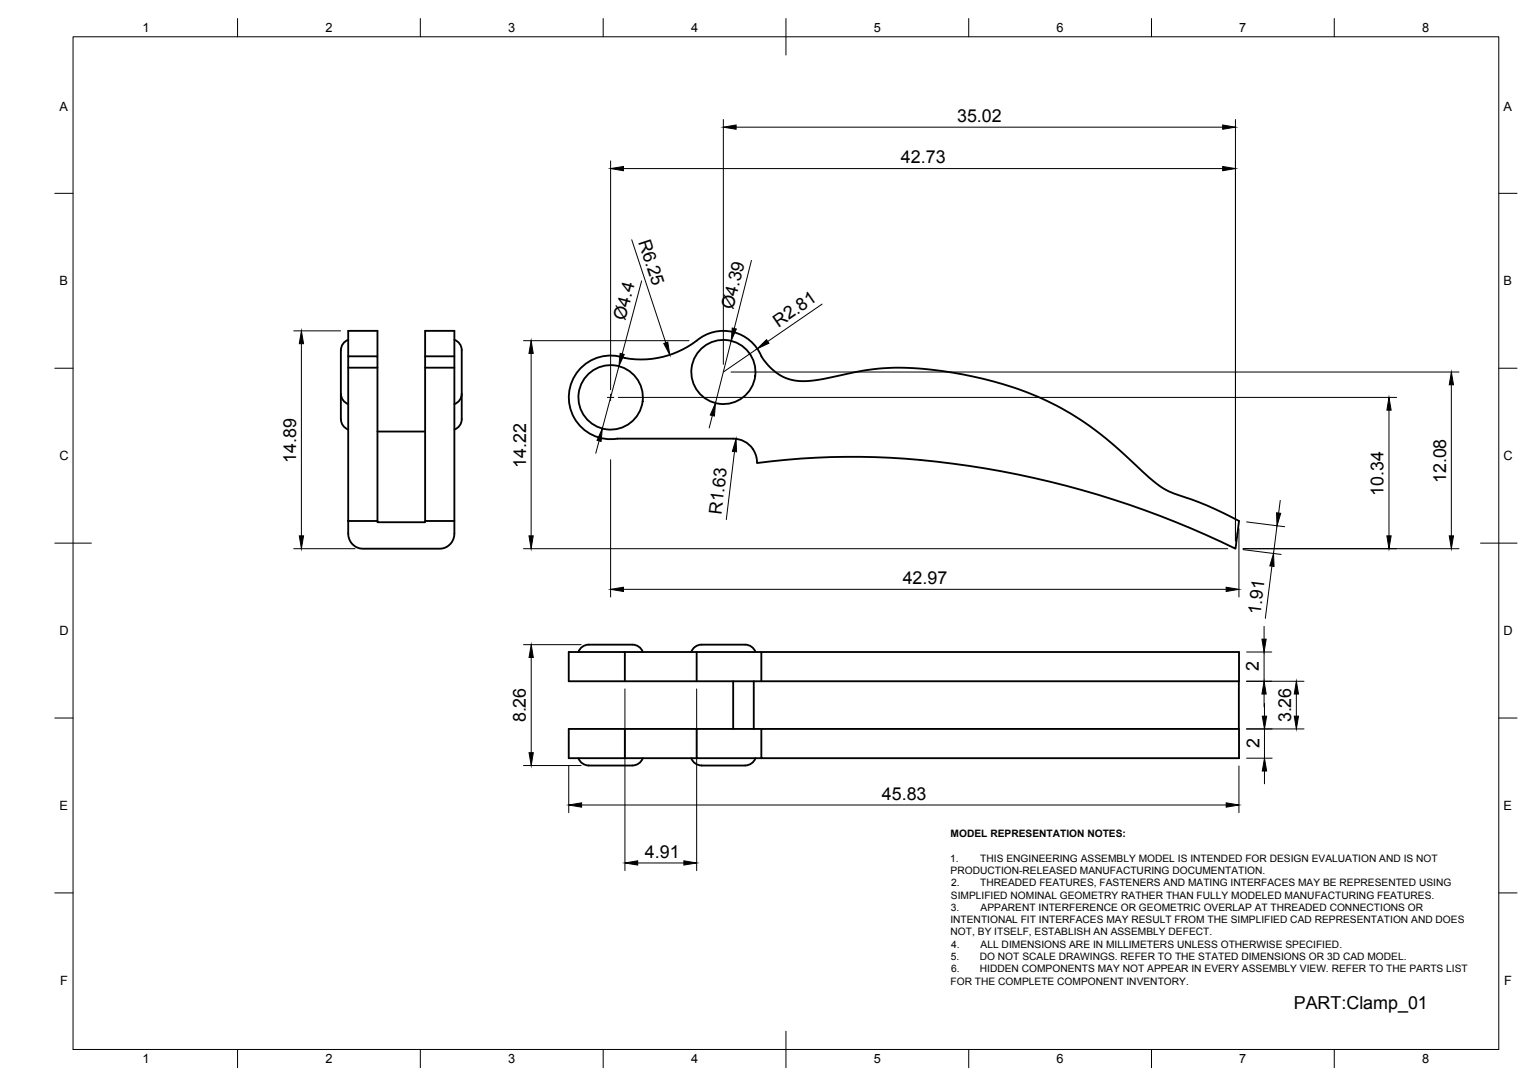
ISO-10303-21;
HEADER;
/* Generated by software containing ST-Developer
 * from STEP Tools, Inc. (www.steptools.com) 
 */

FILE_DESCRIPTION(
/* description */ (''),
/* implementation_level */ '2;1');

FILE_NAME(
/* name */ 'Clamp_01.step',
/* time_stamp */ '2026-10-05T16:20:14-07:00',
/* author */ (''),
/* organization */ (''),
/* preprocessor_version */ 'ST-DEVELOPER v20.2',
/* originating_system */ 'Autodesk Translation Framework v15.15.0.0',
/* authorisation */ '');

FILE_SCHEMA (('AUTOMOTIVE_DESIGN { 1 0 10303 214 3 1 1 }'));
ENDSEC;

DATA;
#10=MECHANICAL_DESIGN_GEOMETRIC_PRESENTATION_REPRESENTATION('',(#253),#23577);
#55=B_SPLINE_SURFACE_WITH_KNOTS('',5,1,((#21755,#21756),(#21757,#21758),
(#21759,#21760),(#21761,#21762),(#21763,#21764),(#21765,#21766),(#21767,
#21768),(#21769,#21770),(#21771,#21772),(#21773,#21774),(#21775,#21776),
(#21777,#21778),(#21779,#21780),(#21781,#21782),(#21783,#21784),(#21785,
#21786),(#21787,#21788),(#21789,#21790),(#21791,#21792),(#21793,#21794),
(#21795,#21796),(#21797,#21798),(#21799,#21800),(#21801,#21802),(#21803,
#21804),(#21805,#21806),(#21807,#21808),(#21809,#21810),(#21811,#21812),
(#21813,#21814),(#21815,#21816),(#21817,#21818),(#21819,#21820),(#21821,
#21822),(#21823,#21824),(#21825,#21826),(#21827,#21828),(#21829,#21830),
(#21831,#21832),(#21833,#21834),(#21835,#21836),(#21837,#21838),(#21839,
#21840),(#21841,#21842),(#21843,#21844),(#21845,#21846),(#21847,#21848),
(#21849,#21850),(#21851,#21852),(#21853,#21854),(#21855,#21856),(#21857,
#21858),(#21859,#21860),(#21861,#21862),(#21863,#21864)),.UNSPECIFIED.,
 .F.,.F.,.F.,(6,1,1,1,1,1,1,1,1,1,1,1,1,1,1,1,1,1,1,1,1,1,1,1,1,1,1,1,1,
1,1,1,1,1,1,1,1,1,1,1,1,1,1,1,1,1,1,1,1,1,6),(2,2),(0.,0.02,0.04,0.06,0.08,
0.1,0.12,0.14,0.16,0.18,0.2,0.22,0.24,0.26,0.28,0.3,0.32,0.34,0.36,0.38,
0.4,0.42,0.44,0.46,0.48,0.5,0.52,0.54,0.56,0.58,0.6,0.62,0.64,0.66,0.68,
0.7,0.72,0.74,0.76,0.78,0.8,0.82,0.84,0.86,0.88,0.9,0.92,0.940000000000001,
0.960000000000001,0.980000000000001,0.99866513431215),(0.,0.24),
 .UNSPECIFIED.);
#56=B_SPLINE_SURFACE_WITH_KNOTS('',5,1,((#22096,#22097),(#22098,#22099),
(#22100,#22101),(#22102,#22103),(#22104,#22105),(#22106,#22107),(#22108,
#22109),(#22110,#22111),(#22112,#22113),(#22114,#22115),(#22116,#22117),
(#22118,#22119),(#22120,#22121),(#22122,#22123),(#22124,#22125),(#22126,
#22127),(#22128,#22129),(#22130,#22131),(#22132,#22133),(#22134,#22135),
(#22136,#22137),(#22138,#22139),(#22140,#22141),(#22142,#22143),(#22144,
#22145),(#22146,#22147),(#22148,#22149),(#22150,#22151),(#22152,#22153),
(#22154,#22155),(#22156,#22157),(#22158,#22159),(#22160,#22161),(#22162,
#22163),(#22164,#22165),(#22166,#22167),(#22168,#22169),(#22170,#22171),
(#22172,#22173),(#22174,#22175),(#22176,#22177),(#22178,#22179),(#22180,
#22181),(#22182,#22183),(#22184,#22185),(#22186,#22187),(#22188,#22189),
(#22190,#22191),(#22192,#22193),(#22194,#22195),(#22196,#22197),(#22198,
#22199),(#22200,#22201),(#22202,#22203),(#22204,#22205)),.UNSPECIFIED.,
 .F.,.F.,.F.,(6,1,1,1,1,1,1,1,1,1,1,1,1,1,1,1,1,1,1,1,1,1,1,1,1,1,1,1,1,
1,1,1,1,1,1,1,1,1,1,1,1,1,1,1,1,1,1,1,1,1,6),(2,2),(0.,0.02,0.04,0.06,0.08,
0.1,0.12,0.14,0.16,0.18,0.2,0.22,0.24,0.26,0.28,0.3,0.32,0.34,0.36,0.38,
0.4,0.42,0.44,0.46,0.48,0.5,0.52,0.54,0.56,0.58,0.6,0.62,0.64,0.66,0.68,
0.7,0.72,0.74,0.76,0.78,0.8,0.82,0.84,0.86,0.88,0.9,0.92,0.940000000000001,
0.960000000000001,0.980000000000001,0.99866513431215),(0.,0.24),
 .UNSPECIFIED.);
#173=B_SPLINE_CURVE_WITH_KNOTS('',3,(#21553,#21554,#21555,#21556,#21557,
#21558,#21559,#21560,#21561,#21562),.UNSPECIFIED.,.F.,.F.,(4,2,2,2,4),(0.304370745831088,
0.340749860871315,0.378176848018549,0.416877357705943,0.456616383722292),
 .UNSPECIFIED.);
#174=B_SPLINE_CURVE_WITH_KNOTS('',3,(#21571,#21572,#21573,#21574,#21575,
#21576,#21577,#21578,#21579,#21580,#21581,#21582),.UNSPECIFIED.,.F.,.F.,
(4,2,2,2,2,4),(-0.956034309409163,-0.919797905610199,-0.883592147057887,
-0.844404551538294,-0.805088366243444,-0.793069564297015),.UNSPECIFIED.);
#175=B_SPLINE_CURVE_WITH_KNOTS('',3,(#21606,#21607,#21608,#21609,#21610,
#21611,#21612,#21613,#21614,#21615,#21616,#21617),.UNSPECIFIED.,.F.,.F.,
(4,2,2,2,2,4),(-0.793069564419585,-0.765429318917777,-0.726356329910807,
-0.690453978752587,-0.655278338273468,-0.628541412295733),.UNSPECIFIED.);
#176=B_SPLINE_CURVE_WITH_KNOTS('',3,(#21620,#21621,#21622,#21623,#21624,
#21625,#21626,#21627,#21628,#21629),.UNSPECIFIED.,.F.,.F.,(4,2,2,2,4),(0.152125107939884,
0.191864133956234,0.230564643643628,0.267991630790861,0.304370745831088),
 .UNSPECIFIED.);
#177=B_SPLINE_CURVE_WITH_KNOTS('',5,(#21645,#21646,#21647,#21648,#21649,
#21650,#21651,#21652,#21653,#21654,#21655,#21656,#21657,#21658,#21659,#21660,
#21661,#21662,#21663,#21664,#21665,#21666,#21667,#21668,#21669,#21670,#21671,
#21672,#21673,#21674,#21675,#21676,#21677,#21678,#21679,#21680,#21681,#21682,
#21683,#21684,#21685,#21686,#21687,#21688,#21689,#21690,#21691,#21692,#21693,
#21694,#21695,#21696,#21697,#21698,#21699),.UNSPECIFIED.,.F.,.F.,(6,1,1,
1,1,1,1,1,1,1,1,1,1,1,1,1,1,1,1,1,1,1,1,1,1,1,1,1,1,1,1,1,1,1,1,1,1,1,1,
1,1,1,1,1,1,1,1,1,1,1,6),(0.,0.02,0.04,0.06,0.08,0.1,0.12,0.14,0.16,0.18,
0.2,0.22,0.24,0.26,0.28,0.3,0.32,0.34,0.36,0.38,0.4,0.42,0.44,0.46,0.48,
0.5,0.52,0.54,0.56,0.58,0.6,0.62,0.64,0.66,0.68,0.7,0.72,0.74,0.76,0.78,
0.8,0.82,0.84,0.86,0.88,0.9,0.92,0.940000000000001,0.960000000000001,0.980000000000001,
0.99866513431215),.UNSPECIFIED.);
#178=B_SPLINE_CURVE_WITH_KNOTS('',5,(#21867,#21868,#21869,#21870,#21871,
#21872,#21873,#21874,#21875,#21876,#21877,#21878,#21879,#21880,#21881,#21882,
#21883,#21884,#21885,#21886,#21887,#21888,#21889,#21890,#21891,#21892,#21893,
#21894,#21895,#21896,#21897,#21898,#21899,#21900,#21901,#21902,#21903,#21904,
#21905,#21906,#21907,#21908,#21909,#21910,#21911,#21912,#21913,#21914,#21915,
#21916,#21917,#21918,#21919,#21920,#21921),.UNSPECIFIED.,.F.,.F.,(6,1,1,
1,1,1,1,1,1,1,1,1,1,1,1,1,1,1,1,1,1,1,1,1,1,1,1,1,1,1,1,1,1,1,1,1,1,1,1,
1,1,1,1,1,1,1,1,1,1,1,6),(0.,0.02,0.04,0.06,0.08,0.1,0.12,0.14,0.16,0.18,
0.2,0.22,0.24,0.26,0.28,0.3,0.32,0.34,0.36,0.38,0.4,0.42,0.44,0.46,0.48,
0.5,0.52,0.54,0.56,0.58,0.6,0.62,0.64,0.66,0.68,0.7,0.72,0.74,0.76,0.78,
0.8,0.82,0.84,0.86,0.88,0.9,0.92,0.940000000000001,0.960000000000001,0.980000000000001,
0.998665134312151),.UNSPECIFIED.);
#179=B_SPLINE_CURVE_WITH_KNOTS('',5,(#21925,#21926,#21927,#21928,#21929,
#21930,#21931,#21932,#21933,#21934,#21935,#21936,#21937,#21938,#21939,#21940,
#21941,#21942,#21943,#21944,#21945,#21946,#21947,#21948,#21949,#21950,#21951,
#21952,#21953,#21954,#21955,#21956,#21957,#21958,#21959,#21960,#21961,#21962,
#21963,#21964,#21965,#21966,#21967,#21968,#21969,#21970,#21971,#21972,#21973,
#21974,#21975,#21976,#21977,#21978,#21979),.UNSPECIFIED.,.F.,.F.,(6,1,1,
1,1,1,1,1,1,1,1,1,1,1,1,1,1,1,1,1,1,1,1,1,1,1,1,1,1,1,1,1,1,1,1,1,1,1,1,
1,1,1,1,1,1,1,1,1,1,1,6),(0.,0.02,0.04,0.06,0.08,0.1,0.12,0.14,0.16,0.18,
0.2,0.22,0.24,0.26,0.28,0.3,0.32,0.34,0.36,0.38,0.4,0.42,0.44,0.46,0.48,
0.5,0.52,0.54,0.56,0.58,0.6,0.62,0.64,0.66,0.68,0.7,0.72,0.74,0.76,0.78,
0.8,0.82,0.84,0.86,0.88,0.9,0.92,0.940000000000001,0.960000000000001,0.980000000000001,
0.99866513431215),.UNSPECIFIED.);
#180=B_SPLINE_CURVE_WITH_KNOTS('',5,(#22022,#22023,#22024,#22025,#22026,
#22027,#22028,#22029,#22030,#22031,#22032,#22033,#22034,#22035,#22036,#22037,
#22038,#22039,#22040,#22041,#22042,#22043,#22044,#22045,#22046,#22047,#22048,
#22049,#22050,#22051,#22052,#22053,#22054,#22055,#22056,#22057,#22058,#22059,
#22060,#22061,#22062,#22063,#22064,#22065,#22066,#22067,#22068,#22069,#22070,
#22071,#22072,#22073,#22074,#22075,#22076),.UNSPECIFIED.,.F.,.F.,(6,1,1,
1,1,1,1,1,1,1,1,1,1,1,1,1,1,1,1,1,1,1,1,1,1,1,1,1,1,1,1,1,1,1,1,1,1,1,1,
1,1,1,1,1,1,1,1,1,1,1,6),(0.,0.02,0.04,0.06,0.08,0.1,0.12,0.14,0.16,0.18,
0.2,0.22,0.24,0.26,0.28,0.3,0.32,0.34,0.36,0.38,0.4,0.42,0.44,0.46,0.48,
0.5,0.52,0.54,0.56,0.58,0.6,0.62,0.64,0.66,0.68,0.7,0.72,0.74,0.76,0.78,
0.8,0.82,0.84,0.86,0.88,0.9,0.92,0.940000000000001,0.960000000000001,0.980000000000001,
0.998665134312151),.UNSPECIFIED.);
#217=TOROIDAL_SURFACE('',#4486,63.3332952479771,1.);
#218=TOROIDAL_SURFACE('',#4490,50.7730300598816,1.);
#219=TOROIDAL_SURFACE('',#4500,63.3332952479771,1.);
#220=TOROIDAL_SURFACE('',#4503,50.7730300598816,1.);
#221=TOROIDAL_SURFACE('',#4513,1.49422838778107,0.75);
#222=TOROIDAL_SURFACE('',#4519,1.48767572173512,0.75);
#223=TOROIDAL_SURFACE('',#4525,1.49422838778107,0.75);
#224=TOROIDAL_SURFACE('',#4532,1.48767572173512,0.75);
#235=SHAPE_REPRESENTATION_RELATIONSHIP('SRR','None',#23618,#244);
#244=ADVANCED_BREP_SHAPE_REPRESENTATION('',(#262),#23574);
#253=STYLED_ITEM('',(#23668),#262);
#262=MANIFOLD_SOLID_BREP('Body1',#4163);
#286=FACE_BOUND('',#778,.T.);
#287=FACE_BOUND('',#779,.T.);
#288=FACE_BOUND('',#800,.T.);
#289=FACE_BOUND('',#801,.T.);
#290=FACE_BOUND('',#803,.T.);
#291=FACE_BOUND('',#804,.T.);
#292=FACE_BOUND('',#809,.T.);
#293=FACE_BOUND('',#810,.T.);
#361=PLANE('',#4505);
#362=PLANE('',#4511);
#363=PLANE('',#4516);
#364=PLANE('',#4517);
#365=PLANE('',#4522);
#366=PLANE('',#4523);
#367=PLANE('',#4529);
#368=PLANE('',#4530);
#369=PLANE('',#4536);
#370=PLANE('',#4541);
#371=PLANE('',#4551);
#372=PLANE('',#4552);
#373=PLANE('',#4555);
#374=PLANE('',#4560);
#375=PLANE('',#4568);
#376=PLANE('',#4569);
#523=FACE_OUTER_BOUND('',#770,.T.);
#524=FACE_OUTER_BOUND('',#771,.T.);
#525=FACE_OUTER_BOUND('',#772,.T.);
#526=FACE_OUTER_BOUND('',#773,.T.);
#527=FACE_OUTER_BOUND('',#774,.T.);
#528=FACE_OUTER_BOUND('',#775,.T.);
#529=FACE_OUTER_BOUND('',#776,.T.);
#530=FACE_OUTER_BOUND('',#777,.T.);
#531=FACE_OUTER_BOUND('',#780,.T.);
#532=FACE_OUTER_BOUND('',#781,.T.);
#533=FACE_OUTER_BOUND('',#782,.T.);
#534=FACE_OUTER_BOUND('',#783,.T.);
#535=FACE_OUTER_BOUND('',#784,.T.);
#536=FACE_OUTER_BOUND('',#785,.T.);
#537=FACE_OUTER_BOUND('',#786,.T.);
#538=FACE_OUTER_BOUND('',#787,.T.);
#539=FACE_OUTER_BOUND('',#788,.T.);
#540=FACE_OUTER_BOUND('',#789,.T.);
#541=FACE_OUTER_BOUND('',#790,.T.);
#542=FACE_OUTER_BOUND('',#791,.T.);
#543=FACE_OUTER_BOUND('',#792,.T.);
#544=FACE_OUTER_BOUND('',#793,.T.);
#545=FACE_OUTER_BOUND('',#794,.T.);
#546=FACE_OUTER_BOUND('',#795,.T.);
#547=FACE_OUTER_BOUND('',#796,.T.);
#548=FACE_OUTER_BOUND('',#797,.T.);
#549=FACE_OUTER_BOUND('',#798,.T.);
#550=FACE_OUTER_BOUND('',#799,.T.);
#551=FACE_OUTER_BOUND('',#802,.T.);
#552=FACE_OUTER_BOUND('',#805,.T.);
#553=FACE_OUTER_BOUND('',#806,.T.);
#554=FACE_OUTER_BOUND('',#807,.T.);
#555=FACE_OUTER_BOUND('',#808,.T.);
#556=FACE_OUTER_BOUND('',#811,.T.);
#557=FACE_OUTER_BOUND('',#812,.T.);
#558=FACE_OUTER_BOUND('',#813,.T.);
#559=FACE_OUTER_BOUND('',#814,.T.);
#560=FACE_OUTER_BOUND('',#815,.T.);
#561=FACE_OUTER_BOUND('',#816,.T.);
#562=FACE_OUTER_BOUND('',#817,.T.);
#563=FACE_OUTER_BOUND('',#818,.T.);
#770=EDGE_LOOP('',(#3387,#3388,#3389,#3390));
#771=EDGE_LOOP('',(#3391,#3392,#3393,#3394));
#772=EDGE_LOOP('',(#3395,#3396,#3397,#3398));
#773=EDGE_LOOP('',(#3399,#3400,#3401,#3402));
#774=EDGE_LOOP('',(#3403,#3404,#3405,#3406,#3407,#3408,#3409,#3410));
#775=EDGE_LOOP('',(#3411,#3412,#3413,#3414));
#776=EDGE_LOOP('',(#3415,#3416,#3417,#3418));
#777=EDGE_LOOP('',(#3419,#3420,#3421,#3422,#3423,#3424,#3425,#3426,#3427));
#778=EDGE_LOOP('',(#3428));
#779=EDGE_LOOP('',(#3429));
#780=EDGE_LOOP('',(#3430));
#781=EDGE_LOOP('',(#3431,#3432,#3433,#3434));
#782=EDGE_LOOP('',(#3435));
#783=EDGE_LOOP('',(#3436));
#784=EDGE_LOOP('',(#3437,#3438,#3439,#3440));
#785=EDGE_LOOP('',(#3441));
#786=EDGE_LOOP('',(#3442));
#787=EDGE_LOOP('',(#3443,#3444,#3445,#3446));
#788=EDGE_LOOP('',(#3447));
#789=EDGE_LOOP('',(#3448));
#790=EDGE_LOOP('',(#3449,#3450,#3451,#3452));
#791=EDGE_LOOP('',(#3453));
#792=EDGE_LOOP('',(#3454,#3455,#3456,#3457));
#793=EDGE_LOOP('',(#3458,#3459,#3460,#3461));
#794=EDGE_LOOP('',(#3462,#3463,#3464,#3465));
#795=EDGE_LOOP('',(#3466,#3467,#3468,#3469));
#796=EDGE_LOOP('',(#3470,#3471,#3472,#3473));
#797=EDGE_LOOP('',(#3474,#3475,#3476,#3477));
#798=EDGE_LOOP('',(#3478,#3479,#3480,#3481));
#799=EDGE_LOOP('',(#3482,#3483,#3484,#3485,#3486,#3487,#3488,#3489,#3490));
#800=EDGE_LOOP('',(#3491));
#801=EDGE_LOOP('',(#3492));
#802=EDGE_LOOP('',(#3493,#3494,#3495,#3496,#3497,#3498,#3499,#3500,#3501));
#803=EDGE_LOOP('',(#3502));
#804=EDGE_LOOP('',(#3503));
#805=EDGE_LOOP('',(#3504,#3505,#3506,#3507));
#806=EDGE_LOOP('',(#3508,#3509,#3510,#3511));
#807=EDGE_LOOP('',(#3512,#3513,#3514,#3515));
#808=EDGE_LOOP('',(#3516,#3517,#3518,#3519,#3520,#3521,#3522,#3523,#3524));
#809=EDGE_LOOP('',(#3525));
#810=EDGE_LOOP('',(#3526));
#811=EDGE_LOOP('',(#3527,#3528,#3529,#3530));
#812=EDGE_LOOP('',(#3531,#3532,#3533,#3534));
#813=EDGE_LOOP('',(#3535,#3536,#3537,#3538));
#814=EDGE_LOOP('',(#3539,#3540,#3541,#3542,#3543,#3544,#3545,#3546,#3547,
#3548));
#815=EDGE_LOOP('',(#3549,#3550,#3551,#3552));
#816=EDGE_LOOP('',(#3553,#3554,#3555,#3556));
#817=EDGE_LOOP('',(#3557,#3558,#3559,#3560));
#818=EDGE_LOOP('',(#3561,#3562,#3563,#3564));
#1069=LINE('',#21587,#1354);
#1070=LINE('',#21590,#1355);
#1071=LINE('',#21593,#1356);
#1072=LINE('',#21599,#1357);
#1073=LINE('',#21601,#1358);
#1074=LINE('',#21603,#1359);
#1075=LINE('',#21637,#1360);
#1076=LINE('',#21700,#1361);
#1077=LINE('',#21743,#1362);
#1078=LINE('',#21747,#1363);
#1079=LINE('',#21751,#1364);
#1080=LINE('',#21753,#1365);
#1081=LINE('',#21754,#1366);
#1082=LINE('',#21923,#1367);
#1083=LINE('',#21980,#1368);
#1084=LINE('',#21985,#1369);
#1085=LINE('',#21991,#1370);
#1086=LINE('',#21997,#1371);
#1087=LINE('',#22000,#1372);
#1088=LINE('',#22002,#1373);
#1089=LINE('',#22008,#1374);
#1090=LINE('',#22009,#1375);
#1091=LINE('',#22012,#1376);
#1092=LINE('',#22016,#1377);
#1093=LINE('',#22020,#1378);
#1094=LINE('',#22083,#1379);
#1095=LINE('',#22089,#1380);
#1096=LINE('',#22091,#1381);
#1097=LINE('',#22093,#1382);
#1098=LINE('',#22095,#1383);
#1099=LINE('',#22206,#1384);
#1100=LINE('',#22208,#1385);
#1101=LINE('',#22210,#1386);
#1354=VECTOR('',#5316,10.);
#1355=VECTOR('',#5319,10.);
#1356=VECTOR('',#5322,10.);
#1357=VECTOR('',#5329,10.);
#1358=VECTOR('',#5330,10.);
#1359=VECTOR('',#5331,10.);
#1360=VECTOR('',#5346,10.);
#1361=VECTOR('',#5353,10.);
#1362=VECTOR('',#5412,1.69478250292167);
#1363=VECTOR('',#5417,1.70133516896762);
#1364=VECTOR('',#5422,10.);
#1365=VECTOR('',#5423,10.);
#1366=VECTOR('',#5424,10.);
#1367=VECTOR('',#5425,10.);
#1368=VECTOR('',#5426,10.);
#1369=VECTOR('',#5431,10.);
#1370=VECTOR('',#5438,10.);
#1371=VECTOR('',#5449,10.);
#1372=VECTOR('',#5452,10.);
#1373=VECTOR('',#5453,10.);
#1374=VECTOR('',#5460,10.);
#1375=VECTOR('',#5461,10.);
#1376=VECTOR('',#5464,10.);
#1377=VECTOR('',#5469,10.);
#1378=VECTOR('',#5474,10.);
#1379=VECTOR('',#5481,10.);
#1380=VECTOR('',#5488,1.69478250292167);
#1381=VECTOR('',#5491,1.70133516896762);
#1382=VECTOR('',#5494,10.);
#1383=VECTOR('',#5497,10.);
#1384=VECTOR('',#5498,10.);
#1385=VECTOR('',#5501,10.);
#1386=VECTOR('',#5504,10.);
#1536=CIRCLE('',#4487,63.3332952479771);
#1537=CIRCLE('',#4488,1.);
#1538=CIRCLE('',#4489,62.3332952479771);
#1539=CIRCLE('',#4491,49.7730300598817);
#1540=CIRCLE('',#4492,50.7730300598817);
#1541=CIRCLE('',#4494,62.3332952479771);
#1542=CIRCLE('',#4496,49.7730300598817);
#1543=CIRCLE('',#4498,1.6332945980533);
#1544=CIRCLE('',#4499,1.6332945980533);
#1545=CIRCLE('',#4501,1.);
#1546=CIRCLE('',#4502,63.3332952479771);
#1547=CIRCLE('',#4504,50.7730300598817);
#1548=CIRCLE('',#4506,2.8615696413584);
#1549=CIRCLE('',#4507,6.2515148621032);
#1550=CIRCLE('',#4508,2.81236096609945);
#1551=CIRCLE('',#4509,2.19478250292167);
#1552=CIRCLE('',#4510,2.20133516896762);
#1553=CIRCLE('',#4512,1.70133516896762);
#1554=CIRCLE('',#4514,1.49422838778107);
#1555=CIRCLE('',#4515,0.75);
#1556=CIRCLE('',#4518,1.69478250292167);
#1557=CIRCLE('',#4520,1.48767572173512);
#1558=CIRCLE('',#4521,0.75);
#1559=CIRCLE('',#4524,1.70133516896762);
#1560=CIRCLE('',#4526,1.49422838778107);
#1561=CIRCLE('',#4527,0.75);
#1562=CIRCLE('',#4528,2.20133516896762);
#1563=CIRCLE('',#4531,1.69478250292167);
#1564=CIRCLE('',#4533,1.48767572173512);
#1565=CIRCLE('',#4534,0.75);
#1566=CIRCLE('',#4535,2.19478250292167);
#1567=CIRCLE('',#4538,1.69478250292167);
#1568=CIRCLE('',#4540,1.70133516896762);
#1569=CIRCLE('',#4543,2.81236096609945);
#1570=CIRCLE('',#4544,2.81236096609945);
#1571=CIRCLE('',#4546,6.2515148621032);
#1572=CIRCLE('',#4547,6.2515148621032);
#1573=CIRCLE('',#4549,2.8615696413584);
#1574=CIRCLE('',#4550,2.8615696413584);
#1575=CIRCLE('',#4553,64.0604216491307);
#1576=CIRCLE('',#4554,51.5001564610352);
#1577=CIRCLE('',#4557,51.5001564610352);
#1578=CIRCLE('',#4559,64.0604216491307);
#1579=CIRCLE('',#4561,2.81236096609945);
#1580=CIRCLE('',#4562,6.2515148621032);
#1581=CIRCLE('',#4563,2.8615696413584);
#1582=CIRCLE('',#4564,1.69478250292167);
#1583=CIRCLE('',#4565,1.70133516896762);
#1893=VERTEX_POINT('',#21551);
#1894=VERTEX_POINT('',#21552);
#1895=VERTEX_POINT('',#21563);
#1896=VERTEX_POINT('',#21565);
#1897=VERTEX_POINT('',#21569);
#1898=VERTEX_POINT('',#21570);
#1899=VERTEX_POINT('',#21586);
#1900=VERTEX_POINT('',#21588);
#1901=VERTEX_POINT('',#21592);
#1902=VERTEX_POINT('',#21596);
#1903=VERTEX_POINT('',#21598);
#1904=VERTEX_POINT('',#21600);
#1905=VERTEX_POINT('',#21602);
#1906=VERTEX_POINT('',#21604);
#1907=VERTEX_POINT('',#21619);
#1908=VERTEX_POINT('',#21630);
#1909=VERTEX_POINT('',#21636);
#1910=VERTEX_POINT('',#21638);
#1911=VERTEX_POINT('',#21640);
#1912=VERTEX_POINT('',#21642);
#1913=VERTEX_POINT('',#21644);
#1914=VERTEX_POINT('',#21701);
#1915=VERTEX_POINT('',#21703);
#1916=VERTEX_POINT('',#21706);
#1917=VERTEX_POINT('',#21709);
#1918=VERTEX_POINT('',#21714);
#1919=VERTEX_POINT('',#21717);
#1920=VERTEX_POINT('',#21722);
#1921=VERTEX_POINT('',#21725);
#1922=VERTEX_POINT('',#21727);
#1923=VERTEX_POINT('',#21732);
#1924=VERTEX_POINT('',#21735);
#1925=VERTEX_POINT('',#21737);
#1926=VERTEX_POINT('',#21742);
#1927=VERTEX_POINT('',#21746);
#1928=VERTEX_POINT('',#21750);
#1929=VERTEX_POINT('',#21752);
#1930=VERTEX_POINT('',#21865);
#1931=VERTEX_POINT('',#21866);
#1932=VERTEX_POINT('',#21922);
#1933=VERTEX_POINT('',#21924);
#1934=VERTEX_POINT('',#21982);
#1935=VERTEX_POINT('',#21984);
#1936=VERTEX_POINT('',#21988);
#1937=VERTEX_POINT('',#21990);
#1938=VERTEX_POINT('',#21999);
#1939=VERTEX_POINT('',#22001);
#1940=VERTEX_POINT('',#22003);
#1941=VERTEX_POINT('',#22007);
#1942=VERTEX_POINT('',#22011);
#1943=VERTEX_POINT('',#22015);
#1944=VERTEX_POINT('',#22019);
#1945=VERTEX_POINT('',#22021);
#1946=VERTEX_POINT('',#22077);
#1947=VERTEX_POINT('',#22079);
#1948=VERTEX_POINT('',#22081);
#1949=VERTEX_POINT('',#22084);
#1950=VERTEX_POINT('',#22086);
#2410=EDGE_CURVE('',#1893,#1894,#173,.T.);
#2411=EDGE_CURVE('',#1894,#1895,#1536,.T.);
#2412=EDGE_CURVE('',#1895,#1896,#1537,.T.);
#2413=EDGE_CURVE('',#1896,#1893,#1538,.T.);
#2414=EDGE_CURVE('',#1897,#1898,#174,.T.);
#2415=EDGE_CURVE('',#1898,#1896,#1539,.T.);
#2416=EDGE_CURVE('',#1895,#1897,#1540,.T.);
#2417=EDGE_CURVE('',#1896,#1899,#1069,.T.);
#2418=EDGE_CURVE('',#1900,#1899,#1541,.T.);
#2419=EDGE_CURVE('',#1893,#1900,#1070,.T.);
#2420=EDGE_CURVE('',#1898,#1901,#1071,.T.);
#2421=EDGE_CURVE('',#1899,#1901,#1542,.T.);
#2422=EDGE_CURVE('',#1897,#1902,#1543,.T.);
#2423=EDGE_CURVE('',#1903,#1902,#1072,.T.);
#2424=EDGE_CURVE('',#1904,#1903,#1073,.T.);
#2425=EDGE_CURVE('',#1904,#1905,#1074,.T.);
#2426=EDGE_CURVE('',#1906,#1905,#1544,.T.);
#2427=EDGE_CURVE('',#1901,#1906,#175,.T.);
#2428=EDGE_CURVE('',#1907,#1900,#176,.T.);
#2429=EDGE_CURVE('',#1899,#1908,#1545,.T.);
#2430=EDGE_CURVE('',#1908,#1907,#1546,.T.);
#2431=EDGE_CURVE('',#1906,#1908,#1547,.T.);
#2432=EDGE_CURVE('',#1905,#1909,#1075,.T.);
#2433=EDGE_CURVE('',#1909,#1910,#1548,.T.);
#2434=EDGE_CURVE('',#1910,#1911,#1549,.T.);
#2435=EDGE_CURVE('',#1911,#1912,#1550,.T.);
#2436=EDGE_CURVE('',#1912,#1913,#177,.T.);
#2437=EDGE_CURVE('',#1913,#1907,#1076,.T.);
#2438=EDGE_CURVE('',#1914,#1914,#1551,.T.);
#2439=EDGE_CURVE('',#1915,#1915,#1552,.T.);
#2440=EDGE_CURVE('',#1916,#1916,#1553,.T.);
#2441=EDGE_CURVE('',#1917,#1917,#1554,.T.);
#2442=EDGE_CURVE('',#1917,#1915,#1555,.T.);
#2443=EDGE_CURVE('',#1918,#1918,#1556,.T.);
#2444=EDGE_CURVE('',#1919,#1919,#1557,.T.);
#2445=EDGE_CURVE('',#1919,#1914,#1558,.T.);
#2446=EDGE_CURVE('',#1920,#1920,#1559,.T.);
#2447=EDGE_CURVE('',#1921,#1921,#1560,.T.);
#2448=EDGE_CURVE('',#1921,#1922,#1561,.T.);
#2449=EDGE_CURVE('',#1922,#1922,#1562,.T.);
#2450=EDGE_CURVE('',#1923,#1923,#1563,.T.);
#2451=EDGE_CURVE('',#1924,#1924,#1564,.T.);
#2452=EDGE_CURVE('',#1924,#1925,#1565,.T.);
#2453=EDGE_CURVE('',#1925,#1925,#1566,.T.);
#2454=EDGE_CURVE('',#1923,#1926,#1077,.T.);
#2455=EDGE_CURVE('',#1926,#1926,#1567,.T.);
#2456=EDGE_CURVE('',#1920,#1927,#1078,.T.);
#2457=EDGE_CURVE('',#1927,#1927,#1568,.T.);
#2458=EDGE_CURVE('',#1928,#1903,#1079,.T.);
#2459=EDGE_CURVE('',#1902,#1929,#1080,.T.);
#2460=EDGE_CURVE('',#1928,#1929,#1081,.T.);
#2461=EDGE_CURVE('',#1930,#1931,#178,.T.);
#2462=EDGE_CURVE('',#1930,#1932,#1082,.T.);
#2463=EDGE_CURVE('',#1932,#1933,#179,.T.);
#2464=EDGE_CURVE('',#1931,#1933,#1083,.T.);
#2465=EDGE_CURVE('',#1934,#1930,#1569,.T.);
#2466=EDGE_CURVE('',#1934,#1935,#1084,.T.);
#2467=EDGE_CURVE('',#1935,#1932,#1570,.T.);
#2468=EDGE_CURVE('',#1934,#1936,#1571,.T.);
#2469=EDGE_CURVE('',#1936,#1937,#1085,.T.);
#2470=EDGE_CURVE('',#1937,#1935,#1572,.T.);
#2471=EDGE_CURVE('',#1928,#1936,#1573,.T.);
#2472=EDGE_CURVE('',#1929,#1937,#1574,.T.);
#2473=EDGE_CURVE('',#1933,#1894,#1086,.T.);
#2474=EDGE_CURVE('',#1903,#1938,#1087,.T.);
#2475=EDGE_CURVE('',#1939,#1931,#1088,.T.);
#2476=EDGE_CURVE('',#1940,#1939,#1575,.T.);
#2477=EDGE_CURVE('',#1938,#1940,#1576,.T.);
#2478=EDGE_CURVE('',#1941,#1938,#1089,.T.);
#2479=EDGE_CURVE('',#1904,#1941,#1090,.T.);
#2480=EDGE_CURVE('',#1942,#1940,#1091,.T.);
#2481=EDGE_CURVE('',#1941,#1942,#1577,.T.);
#2482=EDGE_CURVE('',#1943,#1939,#1092,.T.);
#2483=EDGE_CURVE('',#1942,#1943,#1578,.T.);
#2484=EDGE_CURVE('',#1943,#1944,#1093,.T.);
#2485=EDGE_CURVE('',#1945,#1944,#180,.T.);
#2486=EDGE_CURVE('',#1946,#1945,#1579,.T.);
#2487=EDGE_CURVE('',#1946,#1947,#1580,.T.);
#2488=EDGE_CURVE('',#1948,#1947,#1581,.T.);
#2489=EDGE_CURVE('',#1948,#1904,#1094,.T.);
#2490=EDGE_CURVE('',#1949,#1949,#1582,.T.);
#2491=EDGE_CURVE('',#1950,#1950,#1583,.T.);
#2492=EDGE_CURVE('',#1949,#1918,#1095,.T.);
#2493=EDGE_CURVE('',#1950,#1916,#1096,.T.);
#2494=EDGE_CURVE('',#1948,#1909,#1097,.T.);
#2495=EDGE_CURVE('',#1944,#1913,#1098,.T.);
#2496=EDGE_CURVE('',#1945,#1912,#1099,.T.);
#2497=EDGE_CURVE('',#1946,#1911,#1100,.T.);
#2498=EDGE_CURVE('',#1947,#1910,#1101,.T.);
#3387=ORIENTED_EDGE('',*,*,#2410,.T.);
#3388=ORIENTED_EDGE('',*,*,#2411,.T.);
#3389=ORIENTED_EDGE('',*,*,#2412,.T.);
#3390=ORIENTED_EDGE('',*,*,#2413,.T.);
#3391=ORIENTED_EDGE('',*,*,#2414,.T.);
#3392=ORIENTED_EDGE('',*,*,#2415,.T.);
#3393=ORIENTED_EDGE('',*,*,#2412,.F.);
#3394=ORIENTED_EDGE('',*,*,#2416,.T.);
#3395=ORIENTED_EDGE('',*,*,#2413,.F.);
#3396=ORIENTED_EDGE('',*,*,#2417,.T.);
#3397=ORIENTED_EDGE('',*,*,#2418,.F.);
#3398=ORIENTED_EDGE('',*,*,#2419,.F.);
#3399=ORIENTED_EDGE('',*,*,#2415,.F.);
#3400=ORIENTED_EDGE('',*,*,#2420,.T.);
#3401=ORIENTED_EDGE('',*,*,#2421,.F.);
#3402=ORIENTED_EDGE('',*,*,#2417,.F.);
#3403=ORIENTED_EDGE('',*,*,#2414,.F.);
#3404=ORIENTED_EDGE('',*,*,#2422,.T.);
#3405=ORIENTED_EDGE('',*,*,#2423,.F.);
#3406=ORIENTED_EDGE('',*,*,#2424,.F.);
#3407=ORIENTED_EDGE('',*,*,#2425,.T.);
#3408=ORIENTED_EDGE('',*,*,#2426,.F.);
#3409=ORIENTED_EDGE('',*,*,#2427,.F.);
#3410=ORIENTED_EDGE('',*,*,#2420,.F.);
#3411=ORIENTED_EDGE('',*,*,#2428,.T.);
#3412=ORIENTED_EDGE('',*,*,#2418,.T.);
#3413=ORIENTED_EDGE('',*,*,#2429,.T.);
#3414=ORIENTED_EDGE('',*,*,#2430,.T.);
#3415=ORIENTED_EDGE('',*,*,#2427,.T.);
#3416=ORIENTED_EDGE('',*,*,#2431,.T.);
#3417=ORIENTED_EDGE('',*,*,#2429,.F.);
#3418=ORIENTED_EDGE('',*,*,#2421,.T.);
#3419=ORIENTED_EDGE('',*,*,#2430,.F.);
#3420=ORIENTED_EDGE('',*,*,#2431,.F.);
#3421=ORIENTED_EDGE('',*,*,#2426,.T.);
#3422=ORIENTED_EDGE('',*,*,#2432,.T.);
#3423=ORIENTED_EDGE('',*,*,#2433,.T.);
#3424=ORIENTED_EDGE('',*,*,#2434,.T.);
#3425=ORIENTED_EDGE('',*,*,#2435,.T.);
#3426=ORIENTED_EDGE('',*,*,#2436,.T.);
#3427=ORIENTED_EDGE('',*,*,#2437,.T.);
#3428=ORIENTED_EDGE('',*,*,#2438,.T.);
#3429=ORIENTED_EDGE('',*,*,#2439,.T.);
#3430=ORIENTED_EDGE('',*,*,#2440,.T.);
#3431=ORIENTED_EDGE('',*,*,#2441,.T.);
#3432=ORIENTED_EDGE('',*,*,#2442,.T.);
#3433=ORIENTED_EDGE('',*,*,#2439,.F.);
#3434=ORIENTED_EDGE('',*,*,#2442,.F.);
#3435=ORIENTED_EDGE('',*,*,#2441,.F.);
#3436=ORIENTED_EDGE('',*,*,#2443,.T.);
#3437=ORIENTED_EDGE('',*,*,#2444,.T.);
#3438=ORIENTED_EDGE('',*,*,#2445,.T.);
#3439=ORIENTED_EDGE('',*,*,#2438,.F.);
#3440=ORIENTED_EDGE('',*,*,#2445,.F.);
#3441=ORIENTED_EDGE('',*,*,#2444,.F.);
#3442=ORIENTED_EDGE('',*,*,#2446,.F.);
#3443=ORIENTED_EDGE('',*,*,#2447,.F.);
#3444=ORIENTED_EDGE('',*,*,#2448,.T.);
#3445=ORIENTED_EDGE('',*,*,#2449,.F.);
#3446=ORIENTED_EDGE('',*,*,#2448,.F.);
#3447=ORIENTED_EDGE('',*,*,#2447,.T.);
#3448=ORIENTED_EDGE('',*,*,#2450,.F.);
#3449=ORIENTED_EDGE('',*,*,#2451,.F.);
#3450=ORIENTED_EDGE('',*,*,#2452,.T.);
#3451=ORIENTED_EDGE('',*,*,#2453,.F.);
#3452=ORIENTED_EDGE('',*,*,#2452,.F.);
#3453=ORIENTED_EDGE('',*,*,#2451,.T.);
#3454=ORIENTED_EDGE('',*,*,#2450,.T.);
#3455=ORIENTED_EDGE('',*,*,#2454,.T.);
#3456=ORIENTED_EDGE('',*,*,#2455,.F.);
#3457=ORIENTED_EDGE('',*,*,#2454,.F.);
#3458=ORIENTED_EDGE('',*,*,#2446,.T.);
#3459=ORIENTED_EDGE('',*,*,#2456,.T.);
#3460=ORIENTED_EDGE('',*,*,#2457,.F.);
#3461=ORIENTED_EDGE('',*,*,#2456,.F.);
#3462=ORIENTED_EDGE('',*,*,#2458,.T.);
#3463=ORIENTED_EDGE('',*,*,#2423,.T.);
#3464=ORIENTED_EDGE('',*,*,#2459,.T.);
#3465=ORIENTED_EDGE('',*,*,#2460,.F.);
#3466=ORIENTED_EDGE('',*,*,#2461,.F.);
#3467=ORIENTED_EDGE('',*,*,#2462,.T.);
#3468=ORIENTED_EDGE('',*,*,#2463,.T.);
#3469=ORIENTED_EDGE('',*,*,#2464,.F.);
#3470=ORIENTED_EDGE('',*,*,#2465,.F.);
#3471=ORIENTED_EDGE('',*,*,#2466,.T.);
#3472=ORIENTED_EDGE('',*,*,#2467,.T.);
#3473=ORIENTED_EDGE('',*,*,#2462,.F.);
#3474=ORIENTED_EDGE('',*,*,#2468,.T.);
#3475=ORIENTED_EDGE('',*,*,#2469,.T.);
#3476=ORIENTED_EDGE('',*,*,#2470,.T.);
#3477=ORIENTED_EDGE('',*,*,#2466,.F.);
#3478=ORIENTED_EDGE('',*,*,#2471,.F.);
#3479=ORIENTED_EDGE('',*,*,#2460,.T.);
#3480=ORIENTED_EDGE('',*,*,#2472,.T.);
#3481=ORIENTED_EDGE('',*,*,#2469,.F.);
#3482=ORIENTED_EDGE('',*,*,#2411,.F.);
#3483=ORIENTED_EDGE('',*,*,#2473,.F.);
#3484=ORIENTED_EDGE('',*,*,#2463,.F.);
#3485=ORIENTED_EDGE('',*,*,#2467,.F.);
#3486=ORIENTED_EDGE('',*,*,#2470,.F.);
#3487=ORIENTED_EDGE('',*,*,#2472,.F.);
#3488=ORIENTED_EDGE('',*,*,#2459,.F.);
#3489=ORIENTED_EDGE('',*,*,#2422,.F.);
#3490=ORIENTED_EDGE('',*,*,#2416,.F.);
#3491=ORIENTED_EDGE('',*,*,#2449,.T.);
#3492=ORIENTED_EDGE('',*,*,#2453,.T.);
#3493=ORIENTED_EDGE('',*,*,#2474,.F.);
#3494=ORIENTED_EDGE('',*,*,#2458,.F.);
#3495=ORIENTED_EDGE('',*,*,#2471,.T.);
#3496=ORIENTED_EDGE('',*,*,#2468,.F.);
#3497=ORIENTED_EDGE('',*,*,#2465,.T.);
#3498=ORIENTED_EDGE('',*,*,#2461,.T.);
#3499=ORIENTED_EDGE('',*,*,#2475,.F.);
#3500=ORIENTED_EDGE('',*,*,#2476,.F.);
#3501=ORIENTED_EDGE('',*,*,#2477,.F.);
#3502=ORIENTED_EDGE('',*,*,#2457,.T.);
#3503=ORIENTED_EDGE('',*,*,#2455,.T.);
#3504=ORIENTED_EDGE('',*,*,#2474,.T.);
#3505=ORIENTED_EDGE('',*,*,#2478,.F.);
#3506=ORIENTED_EDGE('',*,*,#2479,.F.);
#3507=ORIENTED_EDGE('',*,*,#2424,.T.);
#3508=ORIENTED_EDGE('',*,*,#2477,.T.);
#3509=ORIENTED_EDGE('',*,*,#2480,.F.);
#3510=ORIENTED_EDGE('',*,*,#2481,.F.);
#3511=ORIENTED_EDGE('',*,*,#2478,.T.);
#3512=ORIENTED_EDGE('',*,*,#2476,.T.);
#3513=ORIENTED_EDGE('',*,*,#2482,.F.);
#3514=ORIENTED_EDGE('',*,*,#2483,.F.);
#3515=ORIENTED_EDGE('',*,*,#2480,.T.);
#3516=ORIENTED_EDGE('',*,*,#2479,.T.);
#3517=ORIENTED_EDGE('',*,*,#2481,.T.);
#3518=ORIENTED_EDGE('',*,*,#2483,.T.);
#3519=ORIENTED_EDGE('',*,*,#2484,.T.);
#3520=ORIENTED_EDGE('',*,*,#2485,.F.);
#3521=ORIENTED_EDGE('',*,*,#2486,.F.);
#3522=ORIENTED_EDGE('',*,*,#2487,.T.);
#3523=ORIENTED_EDGE('',*,*,#2488,.F.);
#3524=ORIENTED_EDGE('',*,*,#2489,.T.);
#3525=ORIENTED_EDGE('',*,*,#2490,.F.);
#3526=ORIENTED_EDGE('',*,*,#2491,.F.);
#3527=ORIENTED_EDGE('',*,*,#2490,.T.);
#3528=ORIENTED_EDGE('',*,*,#2492,.T.);
#3529=ORIENTED_EDGE('',*,*,#2443,.F.);
#3530=ORIENTED_EDGE('',*,*,#2492,.F.);
#3531=ORIENTED_EDGE('',*,*,#2491,.T.);
#3532=ORIENTED_EDGE('',*,*,#2493,.T.);
#3533=ORIENTED_EDGE('',*,*,#2440,.F.);
#3534=ORIENTED_EDGE('',*,*,#2493,.F.);
#3535=ORIENTED_EDGE('',*,*,#2489,.F.);
#3536=ORIENTED_EDGE('',*,*,#2494,.T.);
#3537=ORIENTED_EDGE('',*,*,#2432,.F.);
#3538=ORIENTED_EDGE('',*,*,#2425,.F.);
#3539=ORIENTED_EDGE('',*,*,#2410,.F.);
#3540=ORIENTED_EDGE('',*,*,#2419,.T.);
#3541=ORIENTED_EDGE('',*,*,#2428,.F.);
#3542=ORIENTED_EDGE('',*,*,#2437,.F.);
#3543=ORIENTED_EDGE('',*,*,#2495,.F.);
#3544=ORIENTED_EDGE('',*,*,#2484,.F.);
#3545=ORIENTED_EDGE('',*,*,#2482,.T.);
#3546=ORIENTED_EDGE('',*,*,#2475,.T.);
#3547=ORIENTED_EDGE('',*,*,#2464,.T.);
#3548=ORIENTED_EDGE('',*,*,#2473,.T.);
#3549=ORIENTED_EDGE('',*,*,#2485,.T.);
#3550=ORIENTED_EDGE('',*,*,#2495,.T.);
#3551=ORIENTED_EDGE('',*,*,#2436,.F.);
#3552=ORIENTED_EDGE('',*,*,#2496,.F.);
#3553=ORIENTED_EDGE('',*,*,#2486,.T.);
#3554=ORIENTED_EDGE('',*,*,#2496,.T.);
#3555=ORIENTED_EDGE('',*,*,#2435,.F.);
#3556=ORIENTED_EDGE('',*,*,#2497,.F.);
#3557=ORIENTED_EDGE('',*,*,#2487,.F.);
#3558=ORIENTED_EDGE('',*,*,#2497,.T.);
#3559=ORIENTED_EDGE('',*,*,#2434,.F.);
#3560=ORIENTED_EDGE('',*,*,#2498,.F.);
#3561=ORIENTED_EDGE('',*,*,#2488,.T.);
#3562=ORIENTED_EDGE('',*,*,#2498,.T.);
#3563=ORIENTED_EDGE('',*,*,#2433,.F.);
#3564=ORIENTED_EDGE('',*,*,#2494,.F.);
#3899=CYLINDRICAL_SURFACE('',#4493,62.3332952479771);
#3900=CYLINDRICAL_SURFACE('',#4495,49.7730300598816);
#3901=CYLINDRICAL_SURFACE('',#4497,1.6332945980533);
#3902=CYLINDRICAL_SURFACE('',#4537,1.69478250292167);
#3903=CYLINDRICAL_SURFACE('',#4539,1.70133516896762);
#3904=CYLINDRICAL_SURFACE('',#4542,2.81236096609945);
#3905=CYLINDRICAL_SURFACE('',#4545,6.2515148621032);
#3906=CYLINDRICAL_SURFACE('',#4548,2.8615696413584);
#3907=CYLINDRICAL_SURFACE('',#4556,51.5001564610352);
#3908=CYLINDRICAL_SURFACE('',#4558,64.0604216491307);
#3909=CYLINDRICAL_SURFACE('',#4566,1.69478250292167);
#3910=CYLINDRICAL_SURFACE('',#4567,1.70133516896762);
#3911=CYLINDRICAL_SURFACE('',#4570,2.81236096609945);
#3912=CYLINDRICAL_SURFACE('',#4571,6.2515148621032);
#3913=CYLINDRICAL_SURFACE('',#4572,2.8615696413584);
#4058=ADVANCED_FACE('',(#523),#217,.T.);
#4059=ADVANCED_FACE('',(#524),#218,.T.);
#4060=ADVANCED_FACE('',(#525),#3899,.F.);
#4061=ADVANCED_FACE('',(#526),#3900,.F.);
#4062=ADVANCED_FACE('',(#527),#3901,.F.);
#4063=ADVANCED_FACE('',(#528),#219,.T.);
#4064=ADVANCED_FACE('',(#529),#220,.T.);
#4065=ADVANCED_FACE('',(#530,#286,#287),#361,.T.);
#4066=ADVANCED_FACE('',(#531),#362,.F.);
#4067=ADVANCED_FACE('',(#532),#221,.T.);
#4068=ADVANCED_FACE('',(#533),#363,.T.);
#4069=ADVANCED_FACE('',(#534),#364,.F.);
#4070=ADVANCED_FACE('',(#535),#222,.T.);
#4071=ADVANCED_FACE('',(#536),#365,.T.);
#4072=ADVANCED_FACE('',(#537),#366,.T.);
#4073=ADVANCED_FACE('',(#538),#223,.T.);
#4074=ADVANCED_FACE('',(#539),#367,.F.);
#4075=ADVANCED_FACE('',(#540),#368,.T.);
#4076=ADVANCED_FACE('',(#541),#224,.T.);
#4077=ADVANCED_FACE('',(#542),#369,.F.);
#4078=ADVANCED_FACE('',(#543),#3902,.F.);
#4079=ADVANCED_FACE('',(#544),#3903,.F.);
#4080=ADVANCED_FACE('',(#545),#370,.F.);
#4081=ADVANCED_FACE('',(#546),#55,.F.);
#4082=ADVANCED_FACE('',(#547),#3904,.T.);
#4083=ADVANCED_FACE('',(#548),#3905,.F.);
#4084=ADVANCED_FACE('',(#549),#3906,.T.);
#4085=ADVANCED_FACE('',(#550,#288,#289),#371,.F.);
#4086=ADVANCED_FACE('',(#551,#290,#291),#372,.T.);
#4087=ADVANCED_FACE('',(#552),#373,.T.);
#4088=ADVANCED_FACE('',(#553),#3907,.T.);
#4089=ADVANCED_FACE('',(#554),#3908,.T.);
#4090=ADVANCED_FACE('',(#555,#292,#293),#374,.F.);
#4091=ADVANCED_FACE('',(#556),#3909,.F.);
#4092=ADVANCED_FACE('',(#557),#3910,.F.);
#4093=ADVANCED_FACE('',(#558),#375,.T.);
#4094=ADVANCED_FACE('',(#559),#376,.T.);
#4095=ADVANCED_FACE('',(#560),#56,.T.);
#4096=ADVANCED_FACE('',(#561),#3911,.T.);
#4097=ADVANCED_FACE('',(#562),#3912,.F.);
#4098=ADVANCED_FACE('',(#563),#3913,.T.);
#4163=CLOSED_SHELL('',(#4058,#4059,#4060,#4061,#4062,#4063,#4064,#4065,
#4066,#4067,#4068,#4069,#4070,#4071,#4072,#4073,#4074,#4075,#4076,#4077,
#4078,#4079,#4080,#4081,#4082,#4083,#4084,#4085,#4086,#4087,#4088,#4089,
#4090,#4091,#4092,#4093,#4094,#4095,#4096,#4097,#4098));
#4485=AXIS2_PLACEMENT_3D('',#21549,#5298,#5299);
#4486=AXIS2_PLACEMENT_3D('',#21550,#5300,#5301);
#4487=AXIS2_PLACEMENT_3D('',#21564,#5302,#5303);
#4488=AXIS2_PLACEMENT_3D('',#21566,#5304,#5305);
#4489=AXIS2_PLACEMENT_3D('',#21567,#5306,#5307);
#4490=AXIS2_PLACEMENT_3D('',#21568,#5308,#5309);
#4491=AXIS2_PLACEMENT_3D('',#21583,#5310,#5311);
#4492=AXIS2_PLACEMENT_3D('',#21584,#5312,#5313);
#4493=AXIS2_PLACEMENT_3D('',#21585,#5314,#5315);
#4494=AXIS2_PLACEMENT_3D('',#21589,#5317,#5318);
#4495=AXIS2_PLACEMENT_3D('',#21591,#5320,#5321);
#4496=AXIS2_PLACEMENT_3D('',#21594,#5323,#5324);
#4497=AXIS2_PLACEMENT_3D('',#21595,#5325,#5326);
#4498=AXIS2_PLACEMENT_3D('',#21597,#5327,#5328);
#4499=AXIS2_PLACEMENT_3D('',#21605,#5332,#5333);
#4500=AXIS2_PLACEMENT_3D('',#21618,#5334,#5335);
#4501=AXIS2_PLACEMENT_3D('',#21631,#5336,#5337);
#4502=AXIS2_PLACEMENT_3D('',#21632,#5338,#5339);
#4503=AXIS2_PLACEMENT_3D('',#21633,#5340,#5341);
#4504=AXIS2_PLACEMENT_3D('',#21634,#5342,#5343);
#4505=AXIS2_PLACEMENT_3D('',#21635,#5344,#5345);
#4506=AXIS2_PLACEMENT_3D('',#21639,#5347,#5348);
#4507=AXIS2_PLACEMENT_3D('',#21641,#5349,#5350);
#4508=AXIS2_PLACEMENT_3D('',#21643,#5351,#5352);
#4509=AXIS2_PLACEMENT_3D('',#21702,#5354,#5355);
#4510=AXIS2_PLACEMENT_3D('',#21704,#5356,#5357);
#4511=AXIS2_PLACEMENT_3D('',#21705,#5358,#5359);
#4512=AXIS2_PLACEMENT_3D('',#21707,#5360,#5361);
#4513=AXIS2_PLACEMENT_3D('',#21708,#5362,#5363);
#4514=AXIS2_PLACEMENT_3D('',#21710,#5364,#5365);
#4515=AXIS2_PLACEMENT_3D('',#21711,#5366,#5367);
#4516=AXIS2_PLACEMENT_3D('',#21712,#5368,#5369);
#4517=AXIS2_PLACEMENT_3D('',#21713,#5370,#5371);
#4518=AXIS2_PLACEMENT_3D('',#21715,#5372,#5373);
#4519=AXIS2_PLACEMENT_3D('',#21716,#5374,#5375);
#4520=AXIS2_PLACEMENT_3D('',#21718,#5376,#5377);
#4521=AXIS2_PLACEMENT_3D('',#21719,#5378,#5379);
#4522=AXIS2_PLACEMENT_3D('',#21720,#5380,#5381);
#4523=AXIS2_PLACEMENT_3D('',#21721,#5382,#5383);
#4524=AXIS2_PLACEMENT_3D('',#21723,#5384,#5385);
#4525=AXIS2_PLACEMENT_3D('',#21724,#5386,#5387);
#4526=AXIS2_PLACEMENT_3D('',#21726,#5388,#5389);
#4527=AXIS2_PLACEMENT_3D('',#21728,#5390,#5391);
#4528=AXIS2_PLACEMENT_3D('',#21729,#5392,#5393);
#4529=AXIS2_PLACEMENT_3D('',#21730,#5394,#5395);
#4530=AXIS2_PLACEMENT_3D('',#21731,#5396,#5397);
#4531=AXIS2_PLACEMENT_3D('',#21733,#5398,#5399);
#4532=AXIS2_PLACEMENT_3D('',#21734,#5400,#5401);
#4533=AXIS2_PLACEMENT_3D('',#21736,#5402,#5403);
#4534=AXIS2_PLACEMENT_3D('',#21738,#5404,#5405);
#4535=AXIS2_PLACEMENT_3D('',#21739,#5406,#5407);
#4536=AXIS2_PLACEMENT_3D('',#21740,#5408,#5409);
#4537=AXIS2_PLACEMENT_3D('',#21741,#5410,#5411);
#4538=AXIS2_PLACEMENT_3D('',#21744,#5413,#5414);
#4539=AXIS2_PLACEMENT_3D('',#21745,#5415,#5416);
#4540=AXIS2_PLACEMENT_3D('',#21748,#5418,#5419);
#4541=AXIS2_PLACEMENT_3D('',#21749,#5420,#5421);
#4542=AXIS2_PLACEMENT_3D('',#21981,#5427,#5428);
#4543=AXIS2_PLACEMENT_3D('',#21983,#5429,#5430);
#4544=AXIS2_PLACEMENT_3D('',#21986,#5432,#5433);
#4545=AXIS2_PLACEMENT_3D('',#21987,#5434,#5435);
#4546=AXIS2_PLACEMENT_3D('',#21989,#5436,#5437);
#4547=AXIS2_PLACEMENT_3D('',#21992,#5439,#5440);
#4548=AXIS2_PLACEMENT_3D('',#21993,#5441,#5442);
#4549=AXIS2_PLACEMENT_3D('',#21994,#5443,#5444);
#4550=AXIS2_PLACEMENT_3D('',#21995,#5445,#5446);
#4551=AXIS2_PLACEMENT_3D('',#21996,#5447,#5448);
#4552=AXIS2_PLACEMENT_3D('',#21998,#5450,#5451);
#4553=AXIS2_PLACEMENT_3D('',#22004,#5454,#5455);
#4554=AXIS2_PLACEMENT_3D('',#22005,#5456,#5457);
#4555=AXIS2_PLACEMENT_3D('',#22006,#5458,#5459);
#4556=AXIS2_PLACEMENT_3D('',#22010,#5462,#5463);
#4557=AXIS2_PLACEMENT_3D('',#22013,#5465,#5466);
#4558=AXIS2_PLACEMENT_3D('',#22014,#5467,#5468);
#4559=AXIS2_PLACEMENT_3D('',#22017,#5470,#5471);
#4560=AXIS2_PLACEMENT_3D('',#22018,#5472,#5473);
#4561=AXIS2_PLACEMENT_3D('',#22078,#5475,#5476);
#4562=AXIS2_PLACEMENT_3D('',#22080,#5477,#5478);
#4563=AXIS2_PLACEMENT_3D('',#22082,#5479,#5480);
#4564=AXIS2_PLACEMENT_3D('',#22085,#5482,#5483);
#4565=AXIS2_PLACEMENT_3D('',#22087,#5484,#5485);
#4566=AXIS2_PLACEMENT_3D('',#22088,#5486,#5487);
#4567=AXIS2_PLACEMENT_3D('',#22090,#5489,#5490);
#4568=AXIS2_PLACEMENT_3D('',#22092,#5492,#5493);
#4569=AXIS2_PLACEMENT_3D('',#22094,#5495,#5496);
#4570=AXIS2_PLACEMENT_3D('',#22207,#5499,#5500);
#4571=AXIS2_PLACEMENT_3D('',#22209,#5502,#5503);
#4572=AXIS2_PLACEMENT_3D('',#22211,#5505,#5506);
#5298=DIRECTION('axis',(0.,0.,1.));
#5299=DIRECTION('refdir',(1.,0.,0.));
#5300=DIRECTION('center_axis',(0.,1.,0.));
#5301=DIRECTION('ref_axis',(0.148020831985877,0.,-0.988984243200168));
#5302=DIRECTION('center_axis',(0.,1.,0.));
#5303=DIRECTION('ref_axis',(0.148020831985877,0.,-0.988984243200168));
#5304=DIRECTION('center_axis',(0.999483033337749,0.,-0.0321506775973911));
#5305=DIRECTION('ref_axis',(0.,1.,0.));
#5306=DIRECTION('center_axis',(0.,-1.,0.));
#5307=DIRECTION('ref_axis',(0.148020831985877,0.,-0.988984243200168));
#5308=DIRECTION('center_axis',(0.,1.,0.));
#5309=DIRECTION('ref_axis',(0.,0.,1.));
#5310=DIRECTION('center_axis',(0.,-1.,0.));
#5311=DIRECTION('ref_axis',(-0.143870612043421,0.,-0.989596507163526));
#5312=DIRECTION('center_axis',(0.,1.,0.));
#5313=DIRECTION('ref_axis',(-0.143870612043421,0.,-0.989596507163526));
#5314=DIRECTION('center_axis',(0.,-1.,0.));
#5315=DIRECTION('ref_axis',(-0.0321506775973877,0.,-0.999483033337749));
#5316=DIRECTION('',(0.,-1.,0.));
#5317=DIRECTION('center_axis',(0.,1.,0.));
#5318=DIRECTION('ref_axis',(0.148020831985877,0.,-0.988984243200168));
#5319=DIRECTION('',(0.,-1.,0.));
#5320=DIRECTION('center_axis',(0.,-1.,0.));
#5321=DIRECTION('ref_axis',(-0.253780785521889,0.,-0.967261760279963));
#5322=DIRECTION('',(0.,-1.,0.));
#5323=DIRECTION('center_axis',(0.,1.,0.));
#5324=DIRECTION('ref_axis',(-0.143870612043421,0.,-0.989596507163526));
#5325=DIRECTION('center_axis',(0.,-1.,0.));
#5326=DIRECTION('ref_axis',(-0.125259595502011,0.,-0.992124001188698));
#5327=DIRECTION('center_axis',(0.,1.,0.));
#5328=DIRECTION('ref_axis',(-0.125259595502011,0.,-0.992124001188698));
#5329=DIRECTION('',(0.,1.,0.));
#5330=DIRECTION('',(0.,1.,0.));
#5331=DIRECTION('',(0.,-1.,0.));
#5332=DIRECTION('center_axis',(0.,1.,0.));
#5333=DIRECTION('ref_axis',(-0.125259595502011,0.,-0.992124001188698));
#5334=DIRECTION('center_axis',(0.,1.,0.));
#5335=DIRECTION('ref_axis',(0.148020831985877,0.,-0.988984243200168));
#5336=DIRECTION('center_axis',(0.999483033337749,0.,-0.0321506775973911));
#5337=DIRECTION('ref_axis',(0.0321506775973911,0.,0.999483033337749));
#5338=DIRECTION('center_axis',(0.,-1.,0.));
#5339=DIRECTION('ref_axis',(0.148020831985877,0.,-0.988984243200168));
#5340=DIRECTION('center_axis',(0.,1.,0.));
#5341=DIRECTION('ref_axis',(0.,0.,1.));
#5342=DIRECTION('center_axis',(0.,-1.,0.));
#5343=DIRECTION('ref_axis',(-0.143870612043421,0.,-0.989596507163526));
#5344=DIRECTION('center_axis',(0.,-1.,0.));
#5345=DIRECTION('ref_axis',(-1.,0.,0.));
#5346=DIRECTION('',(-0.992124001188699,0.,0.12525959550201));
#5347=DIRECTION('center_axis',(0.,-1.,0.));
#5348=DIRECTION('ref_axis',(-1.,0.,0.));
#5349=DIRECTION('center_axis',(0.,1.,0.));
#5350=DIRECTION('ref_axis',(0.702611585857253,0.,0.711573579764704));
#5351=DIRECTION('center_axis',(0.,-1.,0.));
#5352=DIRECTION('ref_axis',(-1.,0.,0.));
#5353=DIRECTION('',(0.,0.,1.));
#5354=DIRECTION('center_axis',(0.,1.,0.));
#5355=DIRECTION('ref_axis',(0.,0.,-1.));
#5356=DIRECTION('center_axis',(0.,1.,0.));
#5357=DIRECTION('ref_axis',(0.,0.,-1.));
#5358=DIRECTION('center_axis',(0.,-1.,0.));
#5359=DIRECTION('ref_axis',(1.,0.,0.));
#5360=DIRECTION('center_axis',(0.,1.,0.));
#5361=DIRECTION('ref_axis',(-1.,0.,0.));
#5362=DIRECTION('center_axis',(0.,-1.,0.));
#5363=DIRECTION('ref_axis',(-1.,0.,0.));
#5364=DIRECTION('center_axis',(0.,1.,0.));
#5365=DIRECTION('ref_axis',(-1.,0.,0.));
#5366=DIRECTION('center_axis',(0.,0.,1.));
#5367=DIRECTION('ref_axis',(1.,0.,0.));
#5368=DIRECTION('center_axis',(0.,-1.,0.));
#5369=DIRECTION('ref_axis',(1.,0.,0.));
#5370=DIRECTION('center_axis',(0.,-1.,0.));
#5371=DIRECTION('ref_axis',(1.,0.,0.));
#5372=DIRECTION('center_axis',(0.,1.,0.));
#5373=DIRECTION('ref_axis',(-1.,0.,0.));
#5374=DIRECTION('center_axis',(0.,-1.,0.));
#5375=DIRECTION('ref_axis',(-1.,0.,0.));
#5376=DIRECTION('center_axis',(0.,1.,0.));
#5377=DIRECTION('ref_axis',(-1.,0.,0.));
#5378=DIRECTION('center_axis',(0.,0.,1.));
#5379=DIRECTION('ref_axis',(1.,0.,0.));
#5380=DIRECTION('center_axis',(0.,-1.,0.));
#5381=DIRECTION('ref_axis',(1.,0.,0.));
#5382=DIRECTION('center_axis',(0.,-1.,0.));
#5383=DIRECTION('ref_axis',(1.,0.,0.));
#5384=DIRECTION('center_axis',(0.,1.,0.));
#5385=DIRECTION('ref_axis',(-1.,0.,0.));
#5386=DIRECTION('center_axis',(0.,1.,0.));
#5387=DIRECTION('ref_axis',(-1.,0.,0.));
#5388=DIRECTION('center_axis',(0.,1.,0.));
#5389=DIRECTION('ref_axis',(-1.,0.,0.));
#5390=DIRECTION('center_axis',(0.,0.,-1.));
#5391=DIRECTION('ref_axis',(1.,0.,0.));
#5392=DIRECTION('center_axis',(0.,-1.,0.));
#5393=DIRECTION('ref_axis',(0.,0.,1.));
#5394=DIRECTION('center_axis',(0.,-1.,0.));
#5395=DIRECTION('ref_axis',(1.,0.,0.));
#5396=DIRECTION('center_axis',(0.,-1.,0.));
#5397=DIRECTION('ref_axis',(1.,0.,0.));
#5398=DIRECTION('center_axis',(0.,1.,0.));
#5399=DIRECTION('ref_axis',(-1.,0.,0.));
#5400=DIRECTION('center_axis',(0.,1.,0.));
#5401=DIRECTION('ref_axis',(-1.,0.,0.));
#5402=DIRECTION('center_axis',(0.,1.,0.));
#5403=DIRECTION('ref_axis',(-1.,0.,0.));
#5404=DIRECTION('center_axis',(0.,0.,-1.));
#5405=DIRECTION('ref_axis',(1.,0.,0.));
#5406=DIRECTION('center_axis',(0.,-1.,0.));
#5407=DIRECTION('ref_axis',(0.,0.,1.));
#5408=DIRECTION('center_axis',(0.,-1.,0.));
#5409=DIRECTION('ref_axis',(1.,0.,0.));
#5410=DIRECTION('center_axis',(0.,-1.,0.));
#5411=DIRECTION('ref_axis',(-1.,0.,0.));
#5412=DIRECTION('',(0.,-1.,0.));
#5413=DIRECTION('center_axis',(0.,1.,0.));
#5414=DIRECTION('ref_axis',(-1.,0.,0.));
#5415=DIRECTION('center_axis',(0.,-1.,0.));
#5416=DIRECTION('ref_axis',(-1.,0.,0.));
#5417=DIRECTION('',(0.,-1.,0.));
#5418=DIRECTION('center_axis',(0.,1.,0.));
#5419=DIRECTION('ref_axis',(-1.,0.,0.));
#5420=DIRECTION('center_axis',(-0.12525959550201,0.,-0.992124001188699));
#5421=DIRECTION('ref_axis',(-0.992124001188699,0.,0.12525959550201));
#5422=DIRECTION('',(0.992124001188699,0.,-0.12525959550201));
#5423=DIRECTION('',(-0.992124001188699,0.,0.12525959550201));
#5424=DIRECTION('',(0.,1.,0.));
#5425=DIRECTION('',(0.,1.,0.));
#5426=DIRECTION('',(0.,1.,0.));
#5427=DIRECTION('center_axis',(0.,-1.,0.));
#5428=DIRECTION('ref_axis',(-1.,0.,0.));
#5429=DIRECTION('center_axis',(0.,-1.,0.));
#5430=DIRECTION('ref_axis',(-1.,0.,0.));
#5431=DIRECTION('',(0.,1.,0.));
#5432=DIRECTION('center_axis',(0.,-1.,0.));
#5433=DIRECTION('ref_axis',(-1.,0.,0.));
#5434=DIRECTION('center_axis',(0.,-1.,0.));
#5435=DIRECTION('ref_axis',(0.702611585857253,0.,0.711573579764704));
#5436=DIRECTION('center_axis',(0.,-1.,0.));
#5437=DIRECTION('ref_axis',(0.702611585857253,0.,0.711573579764704));
#5438=DIRECTION('',(0.,1.,0.));
#5439=DIRECTION('center_axis',(0.,1.,0.));
#5440=DIRECTION('ref_axis',(0.702611585857253,0.,0.711573579764704));
#5441=DIRECTION('center_axis',(0.,-1.,0.));
#5442=DIRECTION('ref_axis',(-1.,0.,0.));
#5443=DIRECTION('center_axis',(0.,-1.,0.));
#5444=DIRECTION('ref_axis',(-1.,0.,0.));
#5445=DIRECTION('center_axis',(0.,-1.,0.));
#5446=DIRECTION('ref_axis',(-1.,0.,0.));
#5447=DIRECTION('center_axis',(0.,-1.,0.));
#5448=DIRECTION('ref_axis',(-1.,0.,0.));
#5449=DIRECTION('',(0.,0.,1.));
#5450=DIRECTION('center_axis',(0.,-1.,0.));
#5451=DIRECTION('ref_axis',(-1.,0.,0.));
#5452=DIRECTION('',(0.987175716907317,0.,-0.159637413999743));
#5453=DIRECTION('',(0.,0.,-1.));
#5454=DIRECTION('center_axis',(0.,-1.,0.));
#5455=DIRECTION('ref_axis',(-0.0321506775973883,0.,-0.999483033337749));
#5456=DIRECTION('center_axis',(0.,-1.,0.));
#5457=DIRECTION('ref_axis',(-0.25378078552189,0.,-0.967261760279963));
#5458=DIRECTION('center_axis',(-0.159637413999743,0.,-0.987175716907317));
#5459=DIRECTION('ref_axis',(-0.987175716907317,0.,0.159637413999743));
#5460=DIRECTION('',(0.,1.,0.));
#5461=DIRECTION('',(0.987175716907317,0.,-0.159637413999743));
#5462=DIRECTION('center_axis',(0.,1.,0.));
#5463=DIRECTION('ref_axis',(-0.25378078552189,0.,-0.967261760279963));
#5464=DIRECTION('',(0.,1.,0.));
#5465=DIRECTION('center_axis',(0.,-1.,0.));
#5466=DIRECTION('ref_axis',(-0.25378078552189,0.,-0.967261760279963));
#5467=DIRECTION('center_axis',(0.,1.,0.));
#5468=DIRECTION('ref_axis',(-0.0321506775973883,0.,-0.999483033337749));
#5469=DIRECTION('',(0.,1.,0.));
#5470=DIRECTION('center_axis',(0.,-1.,0.));
#5471=DIRECTION('ref_axis',(-0.0321506775973883,0.,-0.999483033337749));
#5472=DIRECTION('center_axis',(0.,-1.,0.));
#5473=DIRECTION('ref_axis',(-1.,0.,0.));
#5474=DIRECTION('',(0.,0.,-1.));
#5475=DIRECTION('center_axis',(0.,-1.,0.));
#5476=DIRECTION('ref_axis',(-1.,0.,0.));
#5477=DIRECTION('center_axis',(0.,-1.,0.));
#5478=DIRECTION('ref_axis',(0.702611585857253,0.,0.711573579764704));
#5479=DIRECTION('center_axis',(0.,-1.,0.));
#5480=DIRECTION('ref_axis',(-1.,0.,0.));
#5481=DIRECTION('',(0.992124001188699,0.,-0.12525959550201));
#5482=DIRECTION('center_axis',(0.,1.,0.));
#5483=DIRECTION('ref_axis',(-1.,0.,0.));
#5484=DIRECTION('center_axis',(0.,1.,0.));
#5485=DIRECTION('ref_axis',(-1.,0.,0.));
#5486=DIRECTION('center_axis',(0.,-1.,0.));
#5487=DIRECTION('ref_axis',(-1.,0.,0.));
#5488=DIRECTION('',(0.,-1.,0.));
#5489=DIRECTION('center_axis',(0.,-1.,0.));
#5490=DIRECTION('ref_axis',(-1.,0.,0.));
#5491=DIRECTION('',(0.,-1.,0.));
#5492=DIRECTION('center_axis',(0.12525959550201,0.,0.992124001188699));
#5493=DIRECTION('ref_axis',(-0.992124001188699,0.,0.12525959550201));
#5494=DIRECTION('',(0.,-1.,0.));
#5495=DIRECTION('center_axis',(1.,0.,0.));
#5496=DIRECTION('ref_axis',(0.,0.,1.));
#5497=DIRECTION('',(0.,-1.,0.));
#5498=DIRECTION('',(0.,-1.,0.));
#5499=DIRECTION('center_axis',(0.,-1.,0.));
#5500=DIRECTION('ref_axis',(-1.,0.,0.));
#5501=DIRECTION('',(0.,-1.,0.));
#5502=DIRECTION('center_axis',(0.,-1.,0.));
#5503=DIRECTION('ref_axis',(0.702611585857253,0.,0.711573579764704));
#5504=DIRECTION('',(0.,-1.,0.));
#5505=DIRECTION('center_axis',(0.,-1.,0.));
#5506=DIRECTION('ref_axis',(-1.,0.,0.));
#21549=CARTESIAN_POINT('',(0.,0.,0.));
#21550=CARTESIAN_POINT('Origin',(48.2463073637983,2.63165946910082,69.7993133400953));
#21551=CARTESIAN_POINT('',(68.4030878430531,2.63165946910082,10.8150451223526));
#21552=CARTESIAN_POINT('',(68.4030878430531,3.63165946910082,9.7592393254959));
#21553=CARTESIAN_POINT('Ctrl Pts',(68.4030878430531,2.63165946910082,10.8150451223525));
#21554=CARTESIAN_POINT('Ctrl Pts',(68.4030878430531,2.75292318590158,10.8150451223525));
#21555=CARTESIAN_POINT('Ctrl Pts',(68.4030878430531,2.89541248956616,10.785518210578));
#21556=CARTESIAN_POINT('Ctrl Pts',(68.4030878430531,3.12160772551173,10.6887622121246));
#21557=CARTESIAN_POINT('Ctrl Pts',(68.4030878430531,3.24445614290878,10.6032009112127));
#21558=CARTESIAN_POINT('Ctrl Pts',(68.4030878430531,3.4208720057804,10.4207982530401));
#21559=CARTESIAN_POINT('Ctrl Pts',(68.4030878430531,3.50444108649997,10.2904913846535));
#21560=CARTESIAN_POINT('Ctrl Pts',(68.4030878430531,3.60180286326798,10.0478297006472));
#21561=CARTESIAN_POINT('Ctrl Pts',(68.4030878430531,3.63165946910082,9.89170274555042));
#21562=CARTESIAN_POINT('Ctrl Pts',(68.4030878430531,3.63165946910082,9.75923932549592));
#21563=CARTESIAN_POINT('',(46.2100990071005,3.63165946910082,6.49875929437188));
#21564=CARTESIAN_POINT('Origin',(48.2463073637983,3.63165946910082,69.7993133400953));
#21565=CARTESIAN_POINT('',(46.2422496846979,2.63165946910082,7.49824232770964));
#21566=CARTESIAN_POINT('Origin',(46.2100990071005,2.63165946910082,6.49875929437188));
#21567=CARTESIAN_POINT('Origin',(48.2463073637983,2.63165946910082,69.7993133400953));
#21568=CARTESIAN_POINT('Origin',(47.8424863271981,2.63165946910082,57.2455413903711));
#21569=CARTESIAN_POINT('',(34.7952469924111,3.63165946910083,8.17752607283019));
#21570=CARTESIAN_POINT('',(35.2110476607967,2.63165946910082,9.1019927201825));
#21571=CARTESIAN_POINT('Ctrl Pts',(34.7952469924111,3.63165946910082,8.17752607283017));
#21572=CARTESIAN_POINT('Ctrl Pts',(34.8759799564169,3.63165946910082,8.26626550574801));
#21573=CARTESIAN_POINT('Ctrl Pts',(34.9449983032363,3.61474142049672,8.36195924308515));
#21574=CARTESIAN_POINT('Ctrl Pts',(35.0582831826993,3.53935169168844,8.55821406987691));
#21575=CARTESIAN_POINT('Ctrl Pts',(35.0999567345737,3.48253018537934,8.65414743483824));
#21576=CARTESIAN_POINT('Ctrl Pts',(35.1630116537089,3.32658482415735,8.83595184144993));
#21577=CARTESIAN_POINT('Ctrl Pts',(35.1815579931415,3.22702675024014,8.91709062486395));
#21578=CARTESIAN_POINT('Ctrl Pts',(35.2043257611677,3.00160501814149,9.03961250753693));
#21579=CARTESIAN_POINT('Ctrl Pts',(35.2085733818225,2.87754210657412,9.0797469049714));
#21580=CARTESIAN_POINT('Ctrl Pts',(35.2108030098643,2.71019457520481,9.09967056655112));
#21581=CARTESIAN_POINT('Ctrl Pts',(35.2110476607967,2.67089160721875,9.10199272018252));
#21582=CARTESIAN_POINT('Ctrl Pts',(35.2110476607967,2.63165946910082,9.10199272018252));
#21583=CARTESIAN_POINT('Origin',(47.8424863271981,2.63165946910082,57.2455413903711));
#21584=CARTESIAN_POINT('Origin',(47.8424863271981,3.63165946910082,57.2455413903711));
#21585=CARTESIAN_POINT('Origin',(48.2463073637983,-1.63165946910082,69.7993133400953));
#21586=CARTESIAN_POINT('',(46.2422496846979,-2.63165946910082,7.49824232770964));
#21587=CARTESIAN_POINT('',(46.2422496846979,-1.63165946910082,7.49824232770964));
#21588=CARTESIAN_POINT('',(68.4030878430531,-2.63165946910082,10.8150451223526));
#21589=CARTESIAN_POINT('Origin',(48.2463073637983,-2.63165946910082,69.7993133400953));
#21590=CARTESIAN_POINT('',(68.4030878430531,-1.63165946910082,10.8150451223526));
#21591=CARTESIAN_POINT('Origin',(47.8424863271981,-1.63165946910082,57.2455413903711));
#21592=CARTESIAN_POINT('',(35.2110476607967,-2.63165946910082,9.1019927201825));
#21593=CARTESIAN_POINT('',(35.2110476607967,-1.63165946910082,9.1019927201825));
#21594=CARTESIAN_POINT('Origin',(47.8424863271981,-2.63165946910082,57.2455413903711));
#21595=CARTESIAN_POINT('Origin',(33.5871186320447,-1.63165946910082,9.27665168389945));
#21596=CARTESIAN_POINT('',(33.3825328113569,3.63165946910082,7.65622091215892));
#21597=CARTESIAN_POINT('Origin',(33.5871186320447,3.63165946910082,9.27665168389945));
#21598=CARTESIAN_POINT('',(33.3825328113569,1.63165946910082,7.65622091215892));
#21599=CARTESIAN_POINT('',(33.3825328113569,-1.63165946910082,7.65622091215892));
#21600=CARTESIAN_POINT('',(33.3825328113569,-1.63165946910082,7.65622091215892));
#21601=CARTESIAN_POINT('',(33.3825328113569,-1.63165946910082,7.65622091215892));
#21602=CARTESIAN_POINT('',(33.3825328113569,-3.63165946910082,7.65622091215892));
#21603=CARTESIAN_POINT('',(33.3825328113569,-1.63165946910082,7.65622091215892));
#21604=CARTESIAN_POINT('',(34.7952469924111,-3.63165946910083,8.17752607283019));
#21605=CARTESIAN_POINT('Origin',(33.5871186320447,-3.63165946910082,9.27665168389945));
#21606=CARTESIAN_POINT('Ctrl Pts',(35.2110476607967,-2.63165946910082,9.10199272018252));
#21607=CARTESIAN_POINT('Ctrl Pts',(35.2110476607967,-2.72188359741207,9.10199272018252));
#21608=CARTESIAN_POINT('Ctrl Pts',(35.2098600778781,-2.81173320097753,9.08969048819768));
#21609=CARTESIAN_POINT('Ctrl Pts',(35.2022627780083,-3.02201309856609,9.03140539390586));
#21610=CARTESIAN_POINT('Ctrl Pts',(35.1940414919055,-3.13713858706392,8.97430444925498));
#21611=CARTESIAN_POINT('Ctrl Pts',(35.1597938958569,-3.33127027536278,8.83013309837006));
#21612=CARTESIAN_POINT('Ctrl Pts',(35.1353560110358,-3.41069037668281,8.74720827480345));
#21613=CARTESIAN_POINT('Ctrl Pts',(35.0612832730061,-3.53467292791191,8.56686348527488));
#21614=CARTESIAN_POINT('Ctrl Pts',(35.0133178917238,-3.57786071700438,8.47290631505476));
#21615=CARTESIAN_POINT('Ctrl Pts',(34.9057013358328,-3.62294202580524,8.30910075082814));
#21616=CARTESIAN_POINT('Ctrl Pts',(34.8531835012163,-3.63165946910082,8.24120827501279));
#21617=CARTESIAN_POINT('Ctrl Pts',(34.7952469924111,-3.63165946910082,8.17752607283017));
#21618=CARTESIAN_POINT('Origin',(48.2463073637983,-2.63165946910082,69.7993133400953));
#21619=CARTESIAN_POINT('',(68.4030878430531,-3.63165946910082,9.7592393254959));
#21620=CARTESIAN_POINT('Ctrl Pts',(68.4030878430531,-3.63165946910082,9.75923932549592));
#21621=CARTESIAN_POINT('Ctrl Pts',(68.4030878430531,-3.63165946910082,9.89170274555042));
#21622=CARTESIAN_POINT('Ctrl Pts',(68.4030878430531,-3.60180286326798,10.0478297006472));
#21623=CARTESIAN_POINT('Ctrl Pts',(68.4030878430531,-3.50444108649997,10.2904913846535));
#21624=CARTESIAN_POINT('Ctrl Pts',(68.4030878430531,-3.4208720057804,10.4207982530401));
#21625=CARTESIAN_POINT('Ctrl Pts',(68.4030878430531,-3.24445614290878,10.6032009112127));
#21626=CARTESIAN_POINT('Ctrl Pts',(68.4030878430531,-3.12160772551173,10.6887622121246));
#21627=CARTESIAN_POINT('Ctrl Pts',(68.4030878430531,-2.89541248956616,10.785518210578));
#21628=CARTESIAN_POINT('Ctrl Pts',(68.4030878430531,-2.75292318590158,10.8150451223525));
#21629=CARTESIAN_POINT('Ctrl Pts',(68.4030878430531,-2.63165946910082,10.8150451223525));
#21630=CARTESIAN_POINT('',(46.2100990071005,-3.63165946910082,6.49875929437188));
#21631=CARTESIAN_POINT('Origin',(46.2100990071005,-2.63165946910082,6.49875929437188));
#21632=CARTESIAN_POINT('Origin',(48.2463073637983,-3.63165946910082,69.7993133400953));
#21633=CARTESIAN_POINT('Origin',(47.8424863271981,-2.63165946910082,57.2455413903711));
#21634=CARTESIAN_POINT('Origin',(47.8424863271981,-3.63165946910082,57.2455413903711));
#21635=CARTESIAN_POINT('Origin',(45.1279324444747,-3.63165946910082,5.6095740306375));
#21636=CARTESIAN_POINT('',(25.5295906637922,-3.63165946910082,8.64768604728929));
#21637=CARTESIAN_POINT('',(25.5295906637922,-3.63165946910082,8.64768604728929));
#21638=CARTESIAN_POINT('',(25.3459666144763,-3.63165946910082,3.11371049024365));
#21639=CARTESIAN_POINT('Origin',(24.7143466872546,-3.63165946910082,5.90470262206354));
#21640=CARTESIAN_POINT('',(30.067343367632,-3.63165946910082,1.31927109386626));
#21641=CARTESIAN_POINT('Origin',(25.6749565963595,-3.63165946910082,-3.12914171551276));
#21642=CARTESIAN_POINT('',(34.5886335096989,-3.63165946910082,1.82713536652871));
#21643=CARTESIAN_POINT('Origin',(32.143405418954,-3.63165946910082,3.2164639050219));
#21644=CARTESIAN_POINT('',(68.4030878430531,-3.63165946910082,8.90436665637975));
#21645=CARTESIAN_POINT('Ctrl Pts',(34.5886335096989,-3.63165946910082,1.82713536652871));
#21646=CARTESIAN_POINT('Ctrl Pts',(34.6362092203122,-3.63165946910082,1.88586871178367));
#21647=CARTESIAN_POINT('Ctrl Pts',(34.7347815549813,-3.63165946910082,2.0017194640625));
#21648=CARTESIAN_POINT('Ctrl Pts',(34.8929036972094,-3.63165946910082,2.17064518663626));
#21649=CARTESIAN_POINT('Ctrl Pts',(35.1242660582543,-3.63165946910082,2.38619485268891));
#21650=CARTESIAN_POINT('Ctrl Pts',(35.4484610450702,-3.63165946910082,2.63681988122319));
#21651=CARTESIAN_POINT('Ctrl Pts',(35.8096797219068,-3.63165946910082,2.86110227440431));
#21652=CARTESIAN_POINT('Ctrl Pts',(36.2121827052432,-3.63165946910082,3.0431608239682));
#21653=CARTESIAN_POINT('Ctrl Pts',(36.6605471216616,-3.63165946910082,3.1637619392622));
#21654=CARTESIAN_POINT('Ctrl Pts',(37.1573477919055,-3.63165946910082,3.20674836359645));
#21655=CARTESIAN_POINT('Ctrl Pts',(37.7004983976614,-3.63165946910082,3.16593783342347));
#21656=CARTESIAN_POINT('Ctrl Pts',(38.2821772960432,-3.63165946910082,3.04891646974342));
#21657=CARTESIAN_POINT('Ctrl Pts',(38.8922061650653,-3.63165946910082,2.8717108056677));
#21658=CARTESIAN_POINT('Ctrl Pts',(39.5206820976528,-3.63165946910082,2.655119497821));
#21659=CARTESIAN_POINT('Ctrl Pts',(40.1606960032496,-3.63165946910082,2.42058806459878));
#21660=CARTESIAN_POINT('Ctrl Pts',(40.8115544872912,-3.63165946910082,2.18580974752969));
#21661=CARTESIAN_POINT('Ctrl Pts',(41.4774295553453,-3.63165946910082,1.9643608719398));
#21662=CARTESIAN_POINT('Ctrl Pts',(42.1650261486421,-3.63165946910082,1.76629475930708));
#21663=CARTESIAN_POINT('Ctrl Pts',(42.8815153494359,-3.63165946910082,1.59838107318515));
#21664=CARTESIAN_POINT('Ctrl Pts',(43.6325437023826,-3.63165946910082,1.46450753402197));
#21665=CARTESIAN_POINT('Ctrl Pts',(44.4197406663614,-3.63165946910082,1.36594448830542));
#21666=CARTESIAN_POINT('Ctrl Pts',(45.2407218004933,-3.63165946910082,1.30194849827011));
#21667=CARTESIAN_POINT('Ctrl Pts',(46.0905159507805,-3.63165946910082,1.27053601971253));
#21668=CARTESIAN_POINT('Ctrl Pts',(46.9625249651934,-3.63165946910082,1.26918753879412));
#21669=CARTESIAN_POINT('Ctrl Pts',(47.8497123901009,-3.63165946910082,1.29560818694524));
#21670=CARTESIAN_POINT('Ctrl Pts',(48.745595015671,-3.63165946910082,1.3483918257298));
#21671=CARTESIAN_POINT('Ctrl Pts',(49.6455611586008,-3.63165946910082,1.42790750554685));
#21672=CARTESIAN_POINT('Ctrl Pts',(50.5469014142808,-3.63165946910082,1.53623826938649));
#21673=CARTESIAN_POINT('Ctrl Pts',(51.4480843800216,-3.63165946910082,1.67655609650635));
#21674=CARTESIAN_POINT('Ctrl Pts',(52.348266859532,-3.63165946910082,1.85267033982542));
#21675=CARTESIAN_POINT('Ctrl Pts',(53.2467046577141,-3.63165946910082,2.06850649471347));
#21676=CARTESIAN_POINT('Ctrl Pts',(54.1422176988182,-3.63165946910082,2.32761261079463));
#21677=CARTESIAN_POINT('Ctrl Pts',(55.0326050724517,-3.63165946910082,2.63265678969324));
#21678=CARTESIAN_POINT('Ctrl Pts',(55.9141550877392,-3.63165946910082,2.98491249335729));
#21679=CARTESIAN_POINT('Ctrl Pts',(56.7819405807955,-3.63165946910082,3.3836558364077));
#21680=CARTESIAN_POINT('Ctrl Pts',(57.6300359536437,-3.63165946910082,3.82554246975634));
#21681=CARTESIAN_POINT('Ctrl Pts',(58.4517774296143,-3.63165946910082,4.30403237376386));
#21682=CARTESIAN_POINT('Ctrl Pts',(59.2399671195477,-3.63165946910082,4.80867544303911));
#21683=CARTESIAN_POINT('Ctrl Pts',(59.9871842641414,-3.63165946910082,5.32469977859742));
#21684=CARTESIAN_POINT('Ctrl Pts',(60.6858451039897,-3.63165946910082,5.83183545124052));
#21685=CARTESIAN_POINT('Ctrl Pts',(61.3291075829706,-3.63165946910082,6.30568784052758));
#21686=CARTESIAN_POINT('Ctrl Pts',(61.9129286688635,-3.63165946910082,6.72264590044013));
#21687=CARTESIAN_POINT('Ctrl Pts',(62.4378966914009,-3.63165946910082,7.06401270956655));
#21688=CARTESIAN_POINT('Ctrl Pts',(62.9110626727188,-3.63165946910082,7.32028203996567));
#21689=CARTESIAN_POINT('Ctrl Pts',(63.3480382061253,-3.63165946910082,7.49580221124892));
#21690=CARTESIAN_POINT('Ctrl Pts',(63.7742575841079,-3.63165946910082,7.61203807956635));
#21691=CARTESIAN_POINT('Ctrl Pts',(64.2192519841205,-3.63165946910082,7.69914552267219));
#21692=CARTESIAN_POINT('Ctrl Pts',(64.712086468945,-3.63165946910082,7.78936630198725));
#21693=CARTESIAN_POINT('Ctrl Pts',(65.2754113430736,-3.63165946910082,7.90844857460236));
#21694=CARTESIAN_POINT('Ctrl Pts',(65.9237039528771,-3.63165946910082,8.07283920347654));
#21695=CARTESIAN_POINT('Ctrl Pts',(66.6557369297143,-3.63165946910082,8.28958012503506));
#21696=CARTESIAN_POINT('Ctrl Pts',(67.3150092482541,-3.63165946910082,8.50886642156035));
#21697=CARTESIAN_POINT('Ctrl Pts',(67.8492602326033,-3.63165946910082,8.69890399191606));
#21698=CARTESIAN_POINT('Ctrl Pts',(68.2198703338295,-3.63165946910082,8.83566471550562));
#21699=CARTESIAN_POINT('Ctrl Pts',(68.403087843053,-3.63165946910082,8.90436665637972));
#21700=CARTESIAN_POINT('',(68.4030878430531,-3.63165946910082,8.99271976196806));
#21701=CARTESIAN_POINT('',(34.3381879218756,-3.63165946910082,3.2164639050219));
#21702=CARTESIAN_POINT('Origin',(32.143405418954,-3.63165946910082,3.2164639050219));
#21703=CARTESIAN_POINT('',(26.9156818562223,-3.63165946910082,5.90470262206354));
#21704=CARTESIAN_POINT('Origin',(24.7143466872546,-3.63165946910082,5.90470262206354));
#21705=CARTESIAN_POINT('Origin',(24.7143466872546,-3.63165946910082,5.90470262206354));
#21706=CARTESIAN_POINT('',(26.4156818562223,-3.63165946910082,5.90470262206354));
#21707=CARTESIAN_POINT('Origin',(24.7143466872546,-3.63165946910082,5.90470262206354));
#21708=CARTESIAN_POINT('Origin',(24.7143466872546,-3.38165946910082,5.90470262206354));
#21709=CARTESIAN_POINT('',(26.2085750750357,-4.13165946910082,5.90470262206354));
#21710=CARTESIAN_POINT('Origin',(24.7143466872546,-4.13165946910082,5.90470262206354));
#21711=CARTESIAN_POINT('Origin',(26.2085750750357,-3.38165946910082,5.90470262206354));
#21712=CARTESIAN_POINT('Origin',(24.7143466872546,-4.13165946910082,5.90470262206354));
#21713=CARTESIAN_POINT('Origin',(32.143405418954,-3.63165946910082,3.2164639050219));
#21714=CARTESIAN_POINT('',(33.8381879218756,-3.63165946910082,3.2164639050219));
#21715=CARTESIAN_POINT('Origin',(32.143405418954,-3.63165946910082,3.2164639050219));
#21716=CARTESIAN_POINT('Origin',(32.143405418954,-3.38165946910082,3.2164639050219));
#21717=CARTESIAN_POINT('',(33.6310811406891,-4.13165946910082,3.2164639050219));
#21718=CARTESIAN_POINT('Origin',(32.143405418954,-4.13165946910082,3.2164639050219));
#21719=CARTESIAN_POINT('Origin',(33.6310811406891,-3.38165946910082,3.2164639050219));
#21720=CARTESIAN_POINT('Origin',(32.143405418954,-4.13165946910082,3.2164639050219));
#21721=CARTESIAN_POINT('Origin',(24.7143466872546,3.63165946910082,5.90470262206354));
#21722=CARTESIAN_POINT('',(26.4156818562223,3.63165946910082,5.90470262206354));
#21723=CARTESIAN_POINT('Origin',(24.7143466872546,3.63165946910082,5.90470262206354));
#21724=CARTESIAN_POINT('Origin',(24.7143466872546,3.38165946910082,5.90470262206354));
#21725=CARTESIAN_POINT('',(26.2085750750357,4.13165946910082,5.90470262206354));
#21726=CARTESIAN_POINT('Origin',(24.7143466872546,4.13165946910082,5.90470262206354));
#21727=CARTESIAN_POINT('',(26.9156818562223,3.63165946910082,5.90470262206354));
#21728=CARTESIAN_POINT('Origin',(26.2085750750357,3.38165946910082,5.90470262206354));
#21729=CARTESIAN_POINT('Origin',(24.7143466872546,3.63165946910082,5.90470262206354));
#21730=CARTESIAN_POINT('Origin',(24.7143466872546,4.13165946910082,5.90470262206354));
#21731=CARTESIAN_POINT('Origin',(32.143405418954,3.63165946910082,3.2164639050219));
#21732=CARTESIAN_POINT('',(33.8381879218756,3.63165946910082,3.2164639050219));
#21733=CARTESIAN_POINT('Origin',(32.143405418954,3.63165946910082,3.2164639050219));
#21734=CARTESIAN_POINT('Origin',(32.143405418954,3.38165946910082,3.2164639050219));
#21735=CARTESIAN_POINT('',(33.6310811406891,4.13165946910082,3.2164639050219));
#21736=CARTESIAN_POINT('Origin',(32.143405418954,4.13165946910082,3.2164639050219));
#21737=CARTESIAN_POINT('',(34.3381879218756,3.63165946910082,3.2164639050219));
#21738=CARTESIAN_POINT('Origin',(33.6310811406891,3.38165946910082,3.2164639050219));
#21739=CARTESIAN_POINT('Origin',(32.143405418954,3.63165946910082,3.2164639050219));
#21740=CARTESIAN_POINT('Origin',(32.143405418954,4.13165946910082,3.2164639050219));
#21741=CARTESIAN_POINT('Origin',(32.143405418954,1.63165946910082,3.2164639050219));
#21742=CARTESIAN_POINT('',(33.8381879218756,1.63165946910082,3.2164639050219));
#21743=CARTESIAN_POINT('',(33.8381879218757,1.63165946910082,3.2164639050219));
#21744=CARTESIAN_POINT('Origin',(32.143405418954,1.63165946910082,3.2164639050219));
#21745=CARTESIAN_POINT('Origin',(24.7143466872546,1.63165946910082,5.90470262206354));
#21746=CARTESIAN_POINT('',(26.4156818562223,1.63165946910082,5.90470262206354));
#21747=CARTESIAN_POINT('',(26.4156818562222,1.63165946910082,5.90470262206354));
#21748=CARTESIAN_POINT('Origin',(24.7143466872546,1.63165946910082,5.90470262206354));
#21749=CARTESIAN_POINT('Origin',(33.3825328113569,1.63165946910082,7.65622091215892));
#21750=CARTESIAN_POINT('',(25.5295906637922,1.63165946910082,8.64768604728929));
#21751=CARTESIAN_POINT('',(25.5295906637922,1.63165946910082,8.64768604728929));
#21752=CARTESIAN_POINT('',(25.5295906637922,3.63165946910082,8.64768604728929));
#21753=CARTESIAN_POINT('',(25.5295906637922,3.63165946910082,8.64768604728929));
#21754=CARTESIAN_POINT('',(25.5295906637922,1.63165946910082,8.64768604728929));
#21755=CARTESIAN_POINT('Ctrl Pts',(34.5886335096989,1.63165946910082,1.82713536652871));
#21756=CARTESIAN_POINT('Ctrl Pts',(34.5886335096989,4.03165946910082,1.82713536652871));
#21757=CARTESIAN_POINT('Ctrl Pts',(34.6362092203122,1.63165946910082,1.88586871178367));
#21758=CARTESIAN_POINT('Ctrl Pts',(34.6362092203122,4.03165946910082,1.88586871178367));
#21759=CARTESIAN_POINT('Ctrl Pts',(34.7347815549813,1.63165946910082,2.0017194640625));
#21760=CARTESIAN_POINT('Ctrl Pts',(34.7347815549813,4.03165946910082,2.0017194640625));
#21761=CARTESIAN_POINT('Ctrl Pts',(34.8929036972094,1.63165946910082,2.17064518663626));
#21762=CARTESIAN_POINT('Ctrl Pts',(34.8929036972094,4.03165946910082,2.17064518663626));
#21763=CARTESIAN_POINT('Ctrl Pts',(35.1242660582543,1.63165946910082,2.38619485268891));
#21764=CARTESIAN_POINT('Ctrl Pts',(35.1242660582543,4.03165946910082,2.38619485268891));
#21765=CARTESIAN_POINT('Ctrl Pts',(35.4484610450702,1.63165946910082,2.63681988122319));
#21766=CARTESIAN_POINT('Ctrl Pts',(35.4484610450702,4.03165946910082,2.63681988122319));
#21767=CARTESIAN_POINT('Ctrl Pts',(35.8096797219068,1.63165946910082,2.86110227440431));
#21768=CARTESIAN_POINT('Ctrl Pts',(35.8096797219068,4.03165946910082,2.86110227440431));
#21769=CARTESIAN_POINT('Ctrl Pts',(36.2121827052432,1.63165946910082,3.0431608239682));
#21770=CARTESIAN_POINT('Ctrl Pts',(36.2121827052432,4.03165946910082,3.0431608239682));
#21771=CARTESIAN_POINT('Ctrl Pts',(36.6605471216616,1.63165946910082,3.1637619392622));
#21772=CARTESIAN_POINT('Ctrl Pts',(36.6605471216616,4.03165946910082,3.1637619392622));
#21773=CARTESIAN_POINT('Ctrl Pts',(37.1573477919055,1.63165946910082,3.20674836359645));
#21774=CARTESIAN_POINT('Ctrl Pts',(37.1573477919055,4.03165946910082,3.20674836359645));
#21775=CARTESIAN_POINT('Ctrl Pts',(37.7004983976614,1.63165946910082,3.16593783342347));
#21776=CARTESIAN_POINT('Ctrl Pts',(37.7004983976614,4.03165946910082,3.16593783342347));
#21777=CARTESIAN_POINT('Ctrl Pts',(38.2821772960432,1.63165946910082,3.04891646974342));
#21778=CARTESIAN_POINT('Ctrl Pts',(38.2821772960432,4.03165946910082,3.04891646974342));
#21779=CARTESIAN_POINT('Ctrl Pts',(38.8922061650653,1.63165946910082,2.8717108056677));
#21780=CARTESIAN_POINT('Ctrl Pts',(38.8922061650653,4.03165946910082,2.8717108056677));
#21781=CARTESIAN_POINT('Ctrl Pts',(39.5206820976528,1.63165946910082,2.655119497821));
#21782=CARTESIAN_POINT('Ctrl Pts',(39.5206820976528,4.03165946910082,2.655119497821));
#21783=CARTESIAN_POINT('Ctrl Pts',(40.1606960032496,1.63165946910082,2.42058806459878));
#21784=CARTESIAN_POINT('Ctrl Pts',(40.1606960032496,4.03165946910082,2.42058806459878));
#21785=CARTESIAN_POINT('Ctrl Pts',(40.8115544872912,1.63165946910082,2.18580974752969));
#21786=CARTESIAN_POINT('Ctrl Pts',(40.8115544872912,4.03165946910082,2.18580974752969));
#21787=CARTESIAN_POINT('Ctrl Pts',(41.4774295553453,1.63165946910082,1.9643608719398));
#21788=CARTESIAN_POINT('Ctrl Pts',(41.4774295553453,4.03165946910082,1.9643608719398));
#21789=CARTESIAN_POINT('Ctrl Pts',(42.1650261486421,1.63165946910082,1.76629475930708));
#21790=CARTESIAN_POINT('Ctrl Pts',(42.1650261486421,4.03165946910082,1.76629475930708));
#21791=CARTESIAN_POINT('Ctrl Pts',(42.8815153494359,1.63165946910082,1.59838107318515));
#21792=CARTESIAN_POINT('Ctrl Pts',(42.8815153494359,4.03165946910082,1.59838107318515));
#21793=CARTESIAN_POINT('Ctrl Pts',(43.6325437023826,1.63165946910082,1.46450753402197));
#21794=CARTESIAN_POINT('Ctrl Pts',(43.6325437023826,4.03165946910082,1.46450753402197));
#21795=CARTESIAN_POINT('Ctrl Pts',(44.4197406663614,1.63165946910082,1.36594448830542));
#21796=CARTESIAN_POINT('Ctrl Pts',(44.4197406663614,4.03165946910082,1.36594448830542));
#21797=CARTESIAN_POINT('Ctrl Pts',(45.2407218004933,1.63165946910082,1.30194849827011));
#21798=CARTESIAN_POINT('Ctrl Pts',(45.2407218004933,4.03165946910082,1.30194849827011));
#21799=CARTESIAN_POINT('Ctrl Pts',(46.0905159507805,1.63165946910082,1.27053601971253));
#21800=CARTESIAN_POINT('Ctrl Pts',(46.0905159507805,4.03165946910082,1.27053601971253));
#21801=CARTESIAN_POINT('Ctrl Pts',(46.9625249651934,1.63165946910082,1.26918753879412));
#21802=CARTESIAN_POINT('Ctrl Pts',(46.9625249651934,4.03165946910082,1.26918753879412));
#21803=CARTESIAN_POINT('Ctrl Pts',(47.8497123901009,1.63165946910082,1.29560818694524));
#21804=CARTESIAN_POINT('Ctrl Pts',(47.8497123901009,4.03165946910082,1.29560818694524));
#21805=CARTESIAN_POINT('Ctrl Pts',(48.745595015671,1.63165946910082,1.3483918257298));
#21806=CARTESIAN_POINT('Ctrl Pts',(48.745595015671,4.03165946910082,1.3483918257298));
#21807=CARTESIAN_POINT('Ctrl Pts',(49.6455611586008,1.63165946910082,1.42790750554685));
#21808=CARTESIAN_POINT('Ctrl Pts',(49.6455611586008,4.03165946910082,1.42790750554685));
#21809=CARTESIAN_POINT('Ctrl Pts',(50.5469014142808,1.63165946910082,1.53623826938649));
#21810=CARTESIAN_POINT('Ctrl Pts',(50.5469014142808,4.03165946910082,1.53623826938649));
#21811=CARTESIAN_POINT('Ctrl Pts',(51.4480843800216,1.63165946910082,1.67655609650635));
#21812=CARTESIAN_POINT('Ctrl Pts',(51.4480843800216,4.03165946910082,1.67655609650635));
#21813=CARTESIAN_POINT('Ctrl Pts',(52.348266859532,1.63165946910082,1.85267033982542));
#21814=CARTESIAN_POINT('Ctrl Pts',(52.348266859532,4.03165946910082,1.85267033982542));
#21815=CARTESIAN_POINT('Ctrl Pts',(53.2467046577141,1.63165946910082,2.06850649471347));
#21816=CARTESIAN_POINT('Ctrl Pts',(53.2467046577141,4.03165946910082,2.06850649471347));
#21817=CARTESIAN_POINT('Ctrl Pts',(54.1422176988182,1.63165946910082,2.32761261079463));
#21818=CARTESIAN_POINT('Ctrl Pts',(54.1422176988182,4.03165946910082,2.32761261079463));
#21819=CARTESIAN_POINT('Ctrl Pts',(55.0326050724517,1.63165946910082,2.63265678969324));
#21820=CARTESIAN_POINT('Ctrl Pts',(55.0326050724517,4.03165946910082,2.63265678969324));
#21821=CARTESIAN_POINT('Ctrl Pts',(55.9141550877392,1.63165946910082,2.98491249335729));
#21822=CARTESIAN_POINT('Ctrl Pts',(55.9141550877392,4.03165946910082,2.98491249335729));
#21823=CARTESIAN_POINT('Ctrl Pts',(56.7819405807955,1.63165946910082,3.3836558364077));
#21824=CARTESIAN_POINT('Ctrl Pts',(56.7819405807955,4.03165946910082,3.3836558364077));
#21825=CARTESIAN_POINT('Ctrl Pts',(57.6300359536437,1.63165946910082,3.82554246975634));
#21826=CARTESIAN_POINT('Ctrl Pts',(57.6300359536437,4.03165946910082,3.82554246975634));
#21827=CARTESIAN_POINT('Ctrl Pts',(58.4517774296143,1.63165946910082,4.30403237376386));
#21828=CARTESIAN_POINT('Ctrl Pts',(58.4517774296143,4.03165946910082,4.30403237376386));
#21829=CARTESIAN_POINT('Ctrl Pts',(59.2399671195477,1.63165946910082,4.80867544303911));
#21830=CARTESIAN_POINT('Ctrl Pts',(59.2399671195477,4.03165946910082,4.80867544303911));
#21831=CARTESIAN_POINT('Ctrl Pts',(59.9871842641414,1.63165946910082,5.32469977859742));
#21832=CARTESIAN_POINT('Ctrl Pts',(59.9871842641414,4.03165946910082,5.32469977859742));
#21833=CARTESIAN_POINT('Ctrl Pts',(60.6858451039897,1.63165946910082,5.83183545124052));
#21834=CARTESIAN_POINT('Ctrl Pts',(60.6858451039897,4.03165946910082,5.83183545124052));
#21835=CARTESIAN_POINT('Ctrl Pts',(61.3291075829706,1.63165946910082,6.30568784052758));
#21836=CARTESIAN_POINT('Ctrl Pts',(61.3291075829706,4.03165946910082,6.30568784052758));
#21837=CARTESIAN_POINT('Ctrl Pts',(61.9129286688635,1.63165946910082,6.72264590044013));
#21838=CARTESIAN_POINT('Ctrl Pts',(61.9129286688635,4.03165946910082,6.72264590044013));
#21839=CARTESIAN_POINT('Ctrl Pts',(62.4378966914009,1.63165946910082,7.06401270956655));
#21840=CARTESIAN_POINT('Ctrl Pts',(62.4378966914009,4.03165946910082,7.06401270956655));
#21841=CARTESIAN_POINT('Ctrl Pts',(62.9110626727188,1.63165946910082,7.32028203996567));
#21842=CARTESIAN_POINT('Ctrl Pts',(62.9110626727188,4.03165946910082,7.32028203996567));
#21843=CARTESIAN_POINT('Ctrl Pts',(63.3480382061253,1.63165946910082,7.49580221124892));
#21844=CARTESIAN_POINT('Ctrl Pts',(63.3480382061253,4.03165946910082,7.49580221124892));
#21845=CARTESIAN_POINT('Ctrl Pts',(63.7742575841079,1.63165946910082,7.61203807956635));
#21846=CARTESIAN_POINT('Ctrl Pts',(63.7742575841079,4.03165946910082,7.61203807956635));
#21847=CARTESIAN_POINT('Ctrl Pts',(64.2192519841205,1.63165946910082,7.69914552267219));
#21848=CARTESIAN_POINT('Ctrl Pts',(64.2192519841205,4.03165946910082,7.69914552267219));
#21849=CARTESIAN_POINT('Ctrl Pts',(64.712086468945,1.63165946910082,7.78936630198725));
#21850=CARTESIAN_POINT('Ctrl Pts',(64.712086468945,4.03165946910082,7.78936630198725));
#21851=CARTESIAN_POINT('Ctrl Pts',(65.2754113430736,1.63165946910082,7.90844857460236));
#21852=CARTESIAN_POINT('Ctrl Pts',(65.2754113430736,4.03165946910082,7.90844857460236));
#21853=CARTESIAN_POINT('Ctrl Pts',(65.9237039528771,1.63165946910082,8.07283920347654));
#21854=CARTESIAN_POINT('Ctrl Pts',(65.9237039528771,4.03165946910082,8.07283920347654));
#21855=CARTESIAN_POINT('Ctrl Pts',(66.6557369297143,1.63165946910082,8.28958012503506));
#21856=CARTESIAN_POINT('Ctrl Pts',(66.6557369297143,4.03165946910082,8.28958012503506));
#21857=CARTESIAN_POINT('Ctrl Pts',(67.3150092482541,1.63165946910082,8.50886642156035));
#21858=CARTESIAN_POINT('Ctrl Pts',(67.3150092482541,4.03165946910082,8.50886642156035));
#21859=CARTESIAN_POINT('Ctrl Pts',(67.8492602326033,1.63165946910082,8.69890399191606));
#21860=CARTESIAN_POINT('Ctrl Pts',(67.8492602326033,4.03165946910082,8.69890399191606));
#21861=CARTESIAN_POINT('Ctrl Pts',(68.2198703338295,1.63165946910082,8.83566471550562));
#21862=CARTESIAN_POINT('Ctrl Pts',(68.2198703338295,4.03165946910082,8.83566471550562));
#21863=CARTESIAN_POINT('Ctrl Pts',(68.403087843053,1.63165946910082,8.90436665637972));
#21864=CARTESIAN_POINT('Ctrl Pts',(68.403087843053,4.03165946910082,8.90436665637972));
#21865=CARTESIAN_POINT('',(34.5886335096989,1.63165946910082,1.82713536652871));
#21866=CARTESIAN_POINT('',(68.4030878430531,1.63165946910082,8.90436665637975));
#21867=CARTESIAN_POINT('Ctrl Pts',(34.5886335096989,1.63165946910082,1.82713536652871));
#21868=CARTESIAN_POINT('Ctrl Pts',(34.6362092203122,1.63165946910082,1.88586871178367));
#21869=CARTESIAN_POINT('Ctrl Pts',(34.7347815549813,1.63165946910082,2.0017194640625));
#21870=CARTESIAN_POINT('Ctrl Pts',(34.8929036972094,1.63165946910082,2.17064518663626));
#21871=CARTESIAN_POINT('Ctrl Pts',(35.1242660582543,1.63165946910082,2.38619485268891));
#21872=CARTESIAN_POINT('Ctrl Pts',(35.4484610450702,1.63165946910082,2.63681988122319));
#21873=CARTESIAN_POINT('Ctrl Pts',(35.8096797219068,1.63165946910082,2.86110227440431));
#21874=CARTESIAN_POINT('Ctrl Pts',(36.2121827052432,1.63165946910082,3.0431608239682));
#21875=CARTESIAN_POINT('Ctrl Pts',(36.6605471216616,1.63165946910082,3.1637619392622));
#21876=CARTESIAN_POINT('Ctrl Pts',(37.1573477919055,1.63165946910082,3.20674836359645));
#21877=CARTESIAN_POINT('Ctrl Pts',(37.7004983976614,1.63165946910082,3.16593783342347));
#21878=CARTESIAN_POINT('Ctrl Pts',(38.2821772960432,1.63165946910082,3.04891646974342));
#21879=CARTESIAN_POINT('Ctrl Pts',(38.8922061650653,1.63165946910082,2.8717108056677));
#21880=CARTESIAN_POINT('Ctrl Pts',(39.5206820976528,1.63165946910082,2.655119497821));
#21881=CARTESIAN_POINT('Ctrl Pts',(40.1606960032496,1.63165946910082,2.42058806459878));
#21882=CARTESIAN_POINT('Ctrl Pts',(40.8115544872912,1.63165946910082,2.18580974752969));
#21883=CARTESIAN_POINT('Ctrl Pts',(41.4774295553453,1.63165946910082,1.9643608719398));
#21884=CARTESIAN_POINT('Ctrl Pts',(42.1650261486421,1.63165946910082,1.76629475930708));
#21885=CARTESIAN_POINT('Ctrl Pts',(42.8815153494359,1.63165946910082,1.59838107318515));
#21886=CARTESIAN_POINT('Ctrl Pts',(43.6325437023826,1.63165946910082,1.46450753402197));
#21887=CARTESIAN_POINT('Ctrl Pts',(44.4197406663614,1.63165946910082,1.36594448830542));
#21888=CARTESIAN_POINT('Ctrl Pts',(45.2407218004933,1.63165946910082,1.30194849827011));
#21889=CARTESIAN_POINT('Ctrl Pts',(46.0905159507805,1.63165946910082,1.27053601971253));
#21890=CARTESIAN_POINT('Ctrl Pts',(46.9625249651934,1.63165946910082,1.26918753879412));
#21891=CARTESIAN_POINT('Ctrl Pts',(47.8497123901009,1.63165946910082,1.29560818694524));
#21892=CARTESIAN_POINT('Ctrl Pts',(48.745595015671,1.63165946910082,1.3483918257298));
#21893=CARTESIAN_POINT('Ctrl Pts',(49.6455611586008,1.63165946910082,1.42790750554685));
#21894=CARTESIAN_POINT('Ctrl Pts',(50.5469014142808,1.63165946910082,1.53623826938649));
#21895=CARTESIAN_POINT('Ctrl Pts',(51.4480843800216,1.63165946910082,1.67655609650635));
#21896=CARTESIAN_POINT('Ctrl Pts',(52.348266859532,1.63165946910082,1.85267033982542));
#21897=CARTESIAN_POINT('Ctrl Pts',(53.2467046577141,1.63165946910082,2.06850649471347));
#21898=CARTESIAN_POINT('Ctrl Pts',(54.1422176988182,1.63165946910082,2.32761261079463));
#21899=CARTESIAN_POINT('Ctrl Pts',(55.0326050724517,1.63165946910082,2.63265678969324));
#21900=CARTESIAN_POINT('Ctrl Pts',(55.9141550877392,1.63165946910082,2.98491249335729));
#21901=CARTESIAN_POINT('Ctrl Pts',(56.7819405807955,1.63165946910082,3.3836558364077));
#21902=CARTESIAN_POINT('Ctrl Pts',(57.6300359536437,1.63165946910082,3.82554246975634));
#21903=CARTESIAN_POINT('Ctrl Pts',(58.4517774296143,1.63165946910082,4.30403237376386));
#21904=CARTESIAN_POINT('Ctrl Pts',(59.2399671195477,1.63165946910082,4.80867544303911));
#21905=CARTESIAN_POINT('Ctrl Pts',(59.9871842641414,1.63165946910082,5.32469977859742));
#21906=CARTESIAN_POINT('Ctrl Pts',(60.6858451039897,1.63165946910082,5.83183545124052));
#21907=CARTESIAN_POINT('Ctrl Pts',(61.3291075829706,1.63165946910082,6.30568784052758));
#21908=CARTESIAN_POINT('Ctrl Pts',(61.9129286688635,1.63165946910082,6.72264590044013));
#21909=CARTESIAN_POINT('Ctrl Pts',(62.4378966914009,1.63165946910082,7.06401270956655));
#21910=CARTESIAN_POINT('Ctrl Pts',(62.9110626727188,1.63165946910082,7.32028203996567));
#21911=CARTESIAN_POINT('Ctrl Pts',(63.3480382061253,1.63165946910082,7.49580221124892));
#21912=CARTESIAN_POINT('Ctrl Pts',(63.7742575841079,1.63165946910082,7.61203807956635));
#21913=CARTESIAN_POINT('Ctrl Pts',(64.2192519841205,1.63165946910082,7.69914552267219));
#21914=CARTESIAN_POINT('Ctrl Pts',(64.712086468945,1.63165946910082,7.78936630198725));
#21915=CARTESIAN_POINT('Ctrl Pts',(65.2754113430736,1.63165946910082,7.90844857460236));
#21916=CARTESIAN_POINT('Ctrl Pts',(65.9237039528771,1.63165946910082,8.07283920347654));
#21917=CARTESIAN_POINT('Ctrl Pts',(66.6557369297143,1.63165946910082,8.28958012503506));
#21918=CARTESIAN_POINT('Ctrl Pts',(67.3150092482541,1.63165946910082,8.50886642156036));
#21919=CARTESIAN_POINT('Ctrl Pts',(67.8492602326033,1.63165946910082,8.69890399191607));
#21920=CARTESIAN_POINT('Ctrl Pts',(68.2198703338296,1.63165946910082,8.83566471550565));
#21921=CARTESIAN_POINT('Ctrl Pts',(68.4030878430531,1.63165946910082,8.90436665637975));
#21922=CARTESIAN_POINT('',(34.5886335096989,3.63165946910082,1.82713536652871));
#21923=CARTESIAN_POINT('',(34.5886335096989,1.63165946910082,1.82713536652871));
#21924=CARTESIAN_POINT('',(68.4030878430531,3.63165946910082,8.90436665637975));
#21925=CARTESIAN_POINT('Ctrl Pts',(34.5886335096989,3.63165946910082,1.82713536652871));
#21926=CARTESIAN_POINT('Ctrl Pts',(34.6362092203122,3.63165946910082,1.88586871178367));
#21927=CARTESIAN_POINT('Ctrl Pts',(34.7347815549813,3.63165946910082,2.0017194640625));
#21928=CARTESIAN_POINT('Ctrl Pts',(34.8929036972094,3.63165946910082,2.17064518663626));
#21929=CARTESIAN_POINT('Ctrl Pts',(35.1242660582543,3.63165946910082,2.38619485268891));
#21930=CARTESIAN_POINT('Ctrl Pts',(35.4484610450702,3.63165946910082,2.63681988122319));
#21931=CARTESIAN_POINT('Ctrl Pts',(35.8096797219068,3.63165946910082,2.86110227440431));
#21932=CARTESIAN_POINT('Ctrl Pts',(36.2121827052432,3.63165946910082,3.0431608239682));
#21933=CARTESIAN_POINT('Ctrl Pts',(36.6605471216616,3.63165946910082,3.1637619392622));
#21934=CARTESIAN_POINT('Ctrl Pts',(37.1573477919055,3.63165946910082,3.20674836359645));
#21935=CARTESIAN_POINT('Ctrl Pts',(37.7004983976614,3.63165946910082,3.16593783342347));
#21936=CARTESIAN_POINT('Ctrl Pts',(38.2821772960432,3.63165946910082,3.04891646974342));
#21937=CARTESIAN_POINT('Ctrl Pts',(38.8922061650653,3.63165946910082,2.8717108056677));
#21938=CARTESIAN_POINT('Ctrl Pts',(39.5206820976528,3.63165946910082,2.655119497821));
#21939=CARTESIAN_POINT('Ctrl Pts',(40.1606960032496,3.63165946910082,2.42058806459878));
#21940=CARTESIAN_POINT('Ctrl Pts',(40.8115544872912,3.63165946910082,2.18580974752969));
#21941=CARTESIAN_POINT('Ctrl Pts',(41.4774295553453,3.63165946910082,1.9643608719398));
#21942=CARTESIAN_POINT('Ctrl Pts',(42.1650261486421,3.63165946910082,1.76629475930708));
#21943=CARTESIAN_POINT('Ctrl Pts',(42.8815153494359,3.63165946910082,1.59838107318515));
#21944=CARTESIAN_POINT('Ctrl Pts',(43.6325437023826,3.63165946910082,1.46450753402197));
#21945=CARTESIAN_POINT('Ctrl Pts',(44.4197406663614,3.63165946910082,1.36594448830542));
#21946=CARTESIAN_POINT('Ctrl Pts',(45.2407218004933,3.63165946910082,1.30194849827011));
#21947=CARTESIAN_POINT('Ctrl Pts',(46.0905159507805,3.63165946910082,1.27053601971253));
#21948=CARTESIAN_POINT('Ctrl Pts',(46.9625249651934,3.63165946910082,1.26918753879412));
#21949=CARTESIAN_POINT('Ctrl Pts',(47.8497123901009,3.63165946910082,1.29560818694524));
#21950=CARTESIAN_POINT('Ctrl Pts',(48.745595015671,3.63165946910082,1.3483918257298));
#21951=CARTESIAN_POINT('Ctrl Pts',(49.6455611586008,3.63165946910082,1.42790750554685));
#21952=CARTESIAN_POINT('Ctrl Pts',(50.5469014142808,3.63165946910082,1.53623826938649));
#21953=CARTESIAN_POINT('Ctrl Pts',(51.4480843800216,3.63165946910082,1.67655609650635));
#21954=CARTESIAN_POINT('Ctrl Pts',(52.348266859532,3.63165946910082,1.85267033982542));
#21955=CARTESIAN_POINT('Ctrl Pts',(53.2467046577141,3.63165946910082,2.06850649471347));
#21956=CARTESIAN_POINT('Ctrl Pts',(54.1422176988182,3.63165946910082,2.32761261079463));
#21957=CARTESIAN_POINT('Ctrl Pts',(55.0326050724517,3.63165946910082,2.63265678969324));
#21958=CARTESIAN_POINT('Ctrl Pts',(55.9141550877392,3.63165946910082,2.98491249335729));
#21959=CARTESIAN_POINT('Ctrl Pts',(56.7819405807955,3.63165946910082,3.3836558364077));
#21960=CARTESIAN_POINT('Ctrl Pts',(57.6300359536437,3.63165946910082,3.82554246975634));
#21961=CARTESIAN_POINT('Ctrl Pts',(58.4517774296143,3.63165946910082,4.30403237376386));
#21962=CARTESIAN_POINT('Ctrl Pts',(59.2399671195477,3.63165946910082,4.80867544303911));
#21963=CARTESIAN_POINT('Ctrl Pts',(59.9871842641414,3.63165946910082,5.32469977859742));
#21964=CARTESIAN_POINT('Ctrl Pts',(60.6858451039897,3.63165946910082,5.83183545124052));
#21965=CARTESIAN_POINT('Ctrl Pts',(61.3291075829706,3.63165946910082,6.30568784052758));
#21966=CARTESIAN_POINT('Ctrl Pts',(61.9129286688635,3.63165946910082,6.72264590044013));
#21967=CARTESIAN_POINT('Ctrl Pts',(62.4378966914009,3.63165946910082,7.06401270956655));
#21968=CARTESIAN_POINT('Ctrl Pts',(62.9110626727188,3.63165946910082,7.32028203996567));
#21969=CARTESIAN_POINT('Ctrl Pts',(63.3480382061253,3.63165946910082,7.49580221124892));
#21970=CARTESIAN_POINT('Ctrl Pts',(63.7742575841079,3.63165946910082,7.61203807956635));
#21971=CARTESIAN_POINT('Ctrl Pts',(64.2192519841205,3.63165946910082,7.69914552267219));
#21972=CARTESIAN_POINT('Ctrl Pts',(64.712086468945,3.63165946910082,7.78936630198725));
#21973=CARTESIAN_POINT('Ctrl Pts',(65.2754113430736,3.63165946910082,7.90844857460236));
#21974=CARTESIAN_POINT('Ctrl Pts',(65.9237039528771,3.63165946910082,8.07283920347654));
#21975=CARTESIAN_POINT('Ctrl Pts',(66.6557369297143,3.63165946910082,8.28958012503506));
#21976=CARTESIAN_POINT('Ctrl Pts',(67.3150092482541,3.63165946910082,8.50886642156035));
#21977=CARTESIAN_POINT('Ctrl Pts',(67.8492602326033,3.63165946910082,8.69890399191606));
#21978=CARTESIAN_POINT('Ctrl Pts',(68.2198703338295,3.63165946910082,8.83566471550562));
#21979=CARTESIAN_POINT('Ctrl Pts',(68.403087843053,3.63165946910082,8.90436665637972));
#21980=CARTESIAN_POINT('',(68.4030878430531,1.63165946910082,8.90436665637975));
#21981=CARTESIAN_POINT('Origin',(32.143405418954,1.63165946910082,3.2164639050219));
#21982=CARTESIAN_POINT('',(30.067343367632,1.63165946910082,1.31927109386626));
#21983=CARTESIAN_POINT('Origin',(32.143405418954,1.63165946910082,3.2164639050219));
#21984=CARTESIAN_POINT('',(30.067343367632,3.63165946910082,1.31927109386626));
#21985=CARTESIAN_POINT('',(30.067343367632,1.63165946910082,1.31927109386626));
#21986=CARTESIAN_POINT('Origin',(32.143405418954,3.63165946910082,3.2164639050219));
#21987=CARTESIAN_POINT('Origin',(25.6749565963595,1.63165946910082,-3.12914171551276));
#21988=CARTESIAN_POINT('',(25.3459666144763,1.63165946910082,3.11371049024365));
#21989=CARTESIAN_POINT('Origin',(25.6749565963595,1.63165946910082,-3.12914171551276));
#21990=CARTESIAN_POINT('',(25.3459666144763,3.63165946910082,3.11371049024365));
#21991=CARTESIAN_POINT('',(25.3459666144763,1.63165946910082,3.11371049024365));
#21992=CARTESIAN_POINT('Origin',(25.6749565963595,3.63165946910082,-3.12914171551276));
#21993=CARTESIAN_POINT('Origin',(24.7143466872546,1.63165946910082,5.90470262206354));
#21994=CARTESIAN_POINT('Origin',(24.7143466872546,1.63165946910082,5.90470262206354));
#21995=CARTESIAN_POINT('Origin',(24.7143466872546,3.63165946910082,5.90470262206354));
#21996=CARTESIAN_POINT('Origin',(45.1279324444747,3.63165946910082,5.6095740306375));
#21997=CARTESIAN_POINT('',(68.4030878430531,3.63165946910082,8.99271976196806));
#21998=CARTESIAN_POINT('Origin',(45.1279324444747,1.63165946910082,5.6095740306375));
#21999=CARTESIAN_POINT('',(34.7727361660163,1.63165946910082,7.43140939717669));
#22000=CARTESIAN_POINT('',(39.9619395364675,1.63165946910082,6.59225686071356));
#22001=CARTESIAN_POINT('',(68.4030878430531,1.63165946910082,8.99271976196808));
#22002=CARTESIAN_POINT('',(68.4030878430531,1.63165946910082,8.99271976196806));
#22003=CARTESIAN_POINT('',(46.1867214006044,1.63165946910082,5.77200879332694));
#22004=CARTESIAN_POINT('Origin',(48.2463073637983,1.63165946910082,69.7993133400953));
#22005=CARTESIAN_POINT('Origin',(47.8424863271981,1.63165946910082,57.2455413903711));
#22006=CARTESIAN_POINT('Origin',(34.7727361660163,-1.63165946910082,7.43140939717669));
#22007=CARTESIAN_POINT('',(34.7727361660163,-1.63165946910082,7.43140939717669));
#22008=CARTESIAN_POINT('',(34.7727361660163,-1.63165946910082,7.43140939717669));
#22009=CARTESIAN_POINT('',(39.9619395364675,-1.63165946910082,6.59225686071356));
#22010=CARTESIAN_POINT('Origin',(47.8424863271981,-1.63165946910082,57.2455413903711));
#22011=CARTESIAN_POINT('',(46.1867214006044,-1.63165946910082,5.77200879332694));
#22012=CARTESIAN_POINT('',(46.1867214006044,-1.63165946910082,5.77200879332694));
#22013=CARTESIAN_POINT('Origin',(47.8424863271981,-1.63165946910082,57.2455413903711));
#22014=CARTESIAN_POINT('Origin',(48.2463073637983,-1.63165946910082,69.7993133400953));
#22015=CARTESIAN_POINT('',(68.4030878430531,-1.63165946910082,8.99271976196806));
#22016=CARTESIAN_POINT('',(68.4030878430531,-1.63165946910082,8.99271976196806));
#22017=CARTESIAN_POINT('Origin',(48.2463073637983,-1.63165946910082,69.7993133400953));
#22018=CARTESIAN_POINT('Origin',(45.1279324444747,-1.63165946910082,5.6095740306375));
#22019=CARTESIAN_POINT('',(68.4030878430531,-1.63165946910082,8.90436665637975));
#22020=CARTESIAN_POINT('',(68.4030878430531,-1.63165946910082,8.99271976196806));
#22021=CARTESIAN_POINT('',(34.5886335096989,-1.63165946910082,1.82713536652871));
#22022=CARTESIAN_POINT('Ctrl Pts',(34.5886335096989,-1.63165946910082,1.82713536652871));
#22023=CARTESIAN_POINT('Ctrl Pts',(34.6362092203122,-1.63165946910082,1.88586871178367));
#22024=CARTESIAN_POINT('Ctrl Pts',(34.7347815549813,-1.63165946910082,2.0017194640625));
#22025=CARTESIAN_POINT('Ctrl Pts',(34.8929036972094,-1.63165946910082,2.17064518663626));
#22026=CARTESIAN_POINT('Ctrl Pts',(35.1242660582543,-1.63165946910082,2.38619485268891));
#22027=CARTESIAN_POINT('Ctrl Pts',(35.4484610450702,-1.63165946910082,2.63681988122319));
#22028=CARTESIAN_POINT('Ctrl Pts',(35.8096797219068,-1.63165946910082,2.86110227440431));
#22029=CARTESIAN_POINT('Ctrl Pts',(36.2121827052432,-1.63165946910082,3.0431608239682));
#22030=CARTESIAN_POINT('Ctrl Pts',(36.6605471216616,-1.63165946910082,3.1637619392622));
#22031=CARTESIAN_POINT('Ctrl Pts',(37.1573477919055,-1.63165946910082,3.20674836359645));
#22032=CARTESIAN_POINT('Ctrl Pts',(37.7004983976614,-1.63165946910082,3.16593783342347));
#22033=CARTESIAN_POINT('Ctrl Pts',(38.2821772960432,-1.63165946910082,3.04891646974342));
#22034=CARTESIAN_POINT('Ctrl Pts',(38.8922061650653,-1.63165946910082,2.8717108056677));
#22035=CARTESIAN_POINT('Ctrl Pts',(39.5206820976528,-1.63165946910082,2.655119497821));
#22036=CARTESIAN_POINT('Ctrl Pts',(40.1606960032496,-1.63165946910082,2.42058806459878));
#22037=CARTESIAN_POINT('Ctrl Pts',(40.8115544872912,-1.63165946910082,2.18580974752969));
#22038=CARTESIAN_POINT('Ctrl Pts',(41.4774295553453,-1.63165946910082,1.9643608719398));
#22039=CARTESIAN_POINT('Ctrl Pts',(42.1650261486421,-1.63165946910082,1.76629475930708));
#22040=CARTESIAN_POINT('Ctrl Pts',(42.8815153494359,-1.63165946910082,1.59838107318515));
#22041=CARTESIAN_POINT('Ctrl Pts',(43.6325437023826,-1.63165946910082,1.46450753402197));
#22042=CARTESIAN_POINT('Ctrl Pts',(44.4197406663614,-1.63165946910082,1.36594448830542));
#22043=CARTESIAN_POINT('Ctrl Pts',(45.2407218004933,-1.63165946910082,1.30194849827011));
#22044=CARTESIAN_POINT('Ctrl Pts',(46.0905159507805,-1.63165946910082,1.27053601971253));
#22045=CARTESIAN_POINT('Ctrl Pts',(46.9625249651934,-1.63165946910082,1.26918753879412));
#22046=CARTESIAN_POINT('Ctrl Pts',(47.8497123901009,-1.63165946910082,1.29560818694524));
#22047=CARTESIAN_POINT('Ctrl Pts',(48.745595015671,-1.63165946910082,1.3483918257298));
#22048=CARTESIAN_POINT('Ctrl Pts',(49.6455611586008,-1.63165946910082,1.42790750554685));
#22049=CARTESIAN_POINT('Ctrl Pts',(50.5469014142808,-1.63165946910082,1.53623826938649));
#22050=CARTESIAN_POINT('Ctrl Pts',(51.4480843800216,-1.63165946910082,1.67655609650635));
#22051=CARTESIAN_POINT('Ctrl Pts',(52.348266859532,-1.63165946910082,1.85267033982542));
#22052=CARTESIAN_POINT('Ctrl Pts',(53.2467046577141,-1.63165946910082,2.06850649471347));
#22053=CARTESIAN_POINT('Ctrl Pts',(54.1422176988182,-1.63165946910082,2.32761261079463));
#22054=CARTESIAN_POINT('Ctrl Pts',(55.0326050724517,-1.63165946910082,2.63265678969324));
#22055=CARTESIAN_POINT('Ctrl Pts',(55.9141550877392,-1.63165946910082,2.98491249335729));
#22056=CARTESIAN_POINT('Ctrl Pts',(56.7819405807955,-1.63165946910082,3.3836558364077));
#22057=CARTESIAN_POINT('Ctrl Pts',(57.6300359536437,-1.63165946910082,3.82554246975634));
#22058=CARTESIAN_POINT('Ctrl Pts',(58.4517774296143,-1.63165946910082,4.30403237376386));
#22059=CARTESIAN_POINT('Ctrl Pts',(59.2399671195477,-1.63165946910082,4.80867544303911));
#22060=CARTESIAN_POINT('Ctrl Pts',(59.9871842641414,-1.63165946910082,5.32469977859742));
#22061=CARTESIAN_POINT('Ctrl Pts',(60.6858451039897,-1.63165946910082,5.83183545124052));
#22062=CARTESIAN_POINT('Ctrl Pts',(61.3291075829706,-1.63165946910082,6.30568784052758));
#22063=CARTESIAN_POINT('Ctrl Pts',(61.9129286688635,-1.63165946910082,6.72264590044013));
#22064=CARTESIAN_POINT('Ctrl Pts',(62.4378966914009,-1.63165946910082,7.06401270956655));
#22065=CARTESIAN_POINT('Ctrl Pts',(62.9110626727188,-1.63165946910082,7.32028203996567));
#22066=CARTESIAN_POINT('Ctrl Pts',(63.3480382061253,-1.63165946910082,7.49580221124892));
#22067=CARTESIAN_POINT('Ctrl Pts',(63.7742575841079,-1.63165946910082,7.61203807956635));
#22068=CARTESIAN_POINT('Ctrl Pts',(64.2192519841205,-1.63165946910082,7.69914552267219));
#22069=CARTESIAN_POINT('Ctrl Pts',(64.712086468945,-1.63165946910082,7.78936630198725));
#22070=CARTESIAN_POINT('Ctrl Pts',(65.2754113430736,-1.63165946910082,7.90844857460236));
#22071=CARTESIAN_POINT('Ctrl Pts',(65.9237039528771,-1.63165946910082,8.07283920347654));
#22072=CARTESIAN_POINT('Ctrl Pts',(66.6557369297143,-1.63165946910082,8.28958012503506));
#22073=CARTESIAN_POINT('Ctrl Pts',(67.3150092482541,-1.63165946910082,8.50886642156036));
#22074=CARTESIAN_POINT('Ctrl Pts',(67.8492602326033,-1.63165946910082,8.69890399191607));
#22075=CARTESIAN_POINT('Ctrl Pts',(68.2198703338296,-1.63165946910082,8.83566471550565));
#22076=CARTESIAN_POINT('Ctrl Pts',(68.4030878430531,-1.63165946910082,8.90436665637975));
#22077=CARTESIAN_POINT('',(30.067343367632,-1.63165946910082,1.31927109386626));
#22078=CARTESIAN_POINT('Origin',(32.143405418954,-1.63165946910082,3.2164639050219));
#22079=CARTESIAN_POINT('',(25.3459666144763,-1.63165946910082,3.11371049024365));
#22080=CARTESIAN_POINT('Origin',(25.6749565963595,-1.63165946910082,-3.12914171551276));
#22081=CARTESIAN_POINT('',(25.5295906637922,-1.63165946910082,8.64768604728929));
#22082=CARTESIAN_POINT('Origin',(24.7143466872546,-1.63165946910082,5.90470262206354));
#22083=CARTESIAN_POINT('',(25.5295906637922,-1.63165946910082,8.64768604728929));
#22084=CARTESIAN_POINT('',(33.8381879218756,-1.63165946910082,3.2164639050219));
#22085=CARTESIAN_POINT('Origin',(32.143405418954,-1.63165946910082,3.2164639050219));
#22086=CARTESIAN_POINT('',(26.4156818562223,-1.63165946910082,5.90470262206354));
#22087=CARTESIAN_POINT('Origin',(24.7143466872546,-1.63165946910082,5.90470262206354));
#22088=CARTESIAN_POINT('Origin',(32.143405418954,-1.63165946910082,3.2164639050219));
#22089=CARTESIAN_POINT('',(33.8381879218757,-1.63165946910082,3.2164639050219));
#22090=CARTESIAN_POINT('Origin',(24.7143466872546,-1.63165946910082,5.90470262206354));
#22091=CARTESIAN_POINT('',(26.4156818562222,-1.63165946910082,5.90470262206354));
#22092=CARTESIAN_POINT('Origin',(33.3825328113569,-1.63165946910082,7.65622091215892));
#22093=CARTESIAN_POINT('',(25.5295906637922,-1.63165946910082,8.64768604728929));
#22094=CARTESIAN_POINT('Origin',(68.4030878430531,-1.63165946910082,8.90436665637975));
#22095=CARTESIAN_POINT('',(68.4030878430531,-1.63165946910082,8.90436665637975));
#22096=CARTESIAN_POINT('Ctrl Pts',(34.5886335096989,-1.63165946910082,1.82713536652871));
#22097=CARTESIAN_POINT('Ctrl Pts',(34.5886335096989,-4.03165946910082,1.82713536652871));
#22098=CARTESIAN_POINT('Ctrl Pts',(34.6362092203122,-1.63165946910082,1.88586871178367));
#22099=CARTESIAN_POINT('Ctrl Pts',(34.6362092203122,-4.03165946910082,1.88586871178367));
#22100=CARTESIAN_POINT('Ctrl Pts',(34.7347815549813,-1.63165946910082,2.0017194640625));
#22101=CARTESIAN_POINT('Ctrl Pts',(34.7347815549813,-4.03165946910082,2.0017194640625));
#22102=CARTESIAN_POINT('Ctrl Pts',(34.8929036972094,-1.63165946910082,2.17064518663626));
#22103=CARTESIAN_POINT('Ctrl Pts',(34.8929036972094,-4.03165946910082,2.17064518663626));
#22104=CARTESIAN_POINT('Ctrl Pts',(35.1242660582543,-1.63165946910082,2.38619485268891));
#22105=CARTESIAN_POINT('Ctrl Pts',(35.1242660582543,-4.03165946910082,2.38619485268891));
#22106=CARTESIAN_POINT('Ctrl Pts',(35.4484610450702,-1.63165946910082,2.63681988122319));
#22107=CARTESIAN_POINT('Ctrl Pts',(35.4484610450702,-4.03165946910082,2.63681988122319));
#22108=CARTESIAN_POINT('Ctrl Pts',(35.8096797219068,-1.63165946910082,2.86110227440431));
#22109=CARTESIAN_POINT('Ctrl Pts',(35.8096797219068,-4.03165946910082,2.86110227440431));
#22110=CARTESIAN_POINT('Ctrl Pts',(36.2121827052432,-1.63165946910082,3.0431608239682));
#22111=CARTESIAN_POINT('Ctrl Pts',(36.2121827052432,-4.03165946910082,3.0431608239682));
#22112=CARTESIAN_POINT('Ctrl Pts',(36.6605471216616,-1.63165946910082,3.1637619392622));
#22113=CARTESIAN_POINT('Ctrl Pts',(36.6605471216616,-4.03165946910082,3.1637619392622));
#22114=CARTESIAN_POINT('Ctrl Pts',(37.1573477919055,-1.63165946910082,3.20674836359645));
#22115=CARTESIAN_POINT('Ctrl Pts',(37.1573477919055,-4.03165946910082,3.20674836359645));
#22116=CARTESIAN_POINT('Ctrl Pts',(37.7004983976614,-1.63165946910082,3.16593783342347));
#22117=CARTESIAN_POINT('Ctrl Pts',(37.7004983976614,-4.03165946910082,3.16593783342347));
#22118=CARTESIAN_POINT('Ctrl Pts',(38.2821772960432,-1.63165946910082,3.04891646974342));
#22119=CARTESIAN_POINT('Ctrl Pts',(38.2821772960432,-4.03165946910082,3.04891646974342));
#22120=CARTESIAN_POINT('Ctrl Pts',(38.8922061650653,-1.63165946910082,2.8717108056677));
#22121=CARTESIAN_POINT('Ctrl Pts',(38.8922061650653,-4.03165946910082,2.8717108056677));
#22122=CARTESIAN_POINT('Ctrl Pts',(39.5206820976528,-1.63165946910082,2.655119497821));
#22123=CARTESIAN_POINT('Ctrl Pts',(39.5206820976528,-4.03165946910082,2.655119497821));
#22124=CARTESIAN_POINT('Ctrl Pts',(40.1606960032496,-1.63165946910082,2.42058806459878));
#22125=CARTESIAN_POINT('Ctrl Pts',(40.1606960032496,-4.03165946910082,2.42058806459878));
#22126=CARTESIAN_POINT('Ctrl Pts',(40.8115544872912,-1.63165946910082,2.18580974752969));
#22127=CARTESIAN_POINT('Ctrl Pts',(40.8115544872912,-4.03165946910082,2.18580974752969));
#22128=CARTESIAN_POINT('Ctrl Pts',(41.4774295553453,-1.63165946910082,1.9643608719398));
#22129=CARTESIAN_POINT('Ctrl Pts',(41.4774295553453,-4.03165946910082,1.9643608719398));
#22130=CARTESIAN_POINT('Ctrl Pts',(42.1650261486421,-1.63165946910082,1.76629475930708));
#22131=CARTESIAN_POINT('Ctrl Pts',(42.1650261486421,-4.03165946910082,1.76629475930708));
#22132=CARTESIAN_POINT('Ctrl Pts',(42.8815153494359,-1.63165946910082,1.59838107318515));
#22133=CARTESIAN_POINT('Ctrl Pts',(42.8815153494359,-4.03165946910082,1.59838107318515));
#22134=CARTESIAN_POINT('Ctrl Pts',(43.6325437023826,-1.63165946910082,1.46450753402197));
#22135=CARTESIAN_POINT('Ctrl Pts',(43.6325437023826,-4.03165946910082,1.46450753402197));
#22136=CARTESIAN_POINT('Ctrl Pts',(44.4197406663614,-1.63165946910082,1.36594448830542));
#22137=CARTESIAN_POINT('Ctrl Pts',(44.4197406663614,-4.03165946910082,1.36594448830542));
#22138=CARTESIAN_POINT('Ctrl Pts',(45.2407218004933,-1.63165946910082,1.30194849827011));
#22139=CARTESIAN_POINT('Ctrl Pts',(45.2407218004933,-4.03165946910082,1.30194849827011));
#22140=CARTESIAN_POINT('Ctrl Pts',(46.0905159507805,-1.63165946910082,1.27053601971253));
#22141=CARTESIAN_POINT('Ctrl Pts',(46.0905159507805,-4.03165946910082,1.27053601971253));
#22142=CARTESIAN_POINT('Ctrl Pts',(46.9625249651934,-1.63165946910082,1.26918753879412));
#22143=CARTESIAN_POINT('Ctrl Pts',(46.9625249651934,-4.03165946910082,1.26918753879412));
#22144=CARTESIAN_POINT('Ctrl Pts',(47.8497123901009,-1.63165946910082,1.29560818694524));
#22145=CARTESIAN_POINT('Ctrl Pts',(47.8497123901009,-4.03165946910082,1.29560818694524));
#22146=CARTESIAN_POINT('Ctrl Pts',(48.745595015671,-1.63165946910082,1.3483918257298));
#22147=CARTESIAN_POINT('Ctrl Pts',(48.745595015671,-4.03165946910082,1.3483918257298));
#22148=CARTESIAN_POINT('Ctrl Pts',(49.6455611586008,-1.63165946910082,1.42790750554685));
#22149=CARTESIAN_POINT('Ctrl Pts',(49.6455611586008,-4.03165946910082,1.42790750554685));
#22150=CARTESIAN_POINT('Ctrl Pts',(50.5469014142808,-1.63165946910082,1.53623826938649));
#22151=CARTESIAN_POINT('Ctrl Pts',(50.5469014142808,-4.03165946910082,1.53623826938649));
#22152=CARTESIAN_POINT('Ctrl Pts',(51.4480843800216,-1.63165946910082,1.67655609650635));
#22153=CARTESIAN_POINT('Ctrl Pts',(51.4480843800216,-4.03165946910082,1.67655609650635));
#22154=CARTESIAN_POINT('Ctrl Pts',(52.348266859532,-1.63165946910082,1.85267033982542));
#22155=CARTESIAN_POINT('Ctrl Pts',(52.348266859532,-4.03165946910082,1.85267033982542));
#22156=CARTESIAN_POINT('Ctrl Pts',(53.2467046577141,-1.63165946910082,2.06850649471347));
#22157=CARTESIAN_POINT('Ctrl Pts',(53.2467046577141,-4.03165946910082,2.06850649471347));
#22158=CARTESIAN_POINT('Ctrl Pts',(54.1422176988182,-1.63165946910082,2.32761261079463));
#22159=CARTESIAN_POINT('Ctrl Pts',(54.1422176988182,-4.03165946910082,2.32761261079463));
#22160=CARTESIAN_POINT('Ctrl Pts',(55.0326050724517,-1.63165946910082,2.63265678969324));
#22161=CARTESIAN_POINT('Ctrl Pts',(55.0326050724517,-4.03165946910082,2.63265678969324));
#22162=CARTESIAN_POINT('Ctrl Pts',(55.9141550877392,-1.63165946910082,2.98491249335729));
#22163=CARTESIAN_POINT('Ctrl Pts',(55.9141550877392,-4.03165946910082,2.98491249335729));
#22164=CARTESIAN_POINT('Ctrl Pts',(56.7819405807955,-1.63165946910082,3.3836558364077));
#22165=CARTESIAN_POINT('Ctrl Pts',(56.7819405807955,-4.03165946910082,3.3836558364077));
#22166=CARTESIAN_POINT('Ctrl Pts',(57.6300359536437,-1.63165946910082,3.82554246975634));
#22167=CARTESIAN_POINT('Ctrl Pts',(57.6300359536437,-4.03165946910082,3.82554246975634));
#22168=CARTESIAN_POINT('Ctrl Pts',(58.4517774296143,-1.63165946910082,4.30403237376386));
#22169=CARTESIAN_POINT('Ctrl Pts',(58.4517774296143,-4.03165946910082,4.30403237376386));
#22170=CARTESIAN_POINT('Ctrl Pts',(59.2399671195477,-1.63165946910082,4.80867544303911));
#22171=CARTESIAN_POINT('Ctrl Pts',(59.2399671195477,-4.03165946910082,4.80867544303911));
#22172=CARTESIAN_POINT('Ctrl Pts',(59.9871842641414,-1.63165946910082,5.32469977859742));
#22173=CARTESIAN_POINT('Ctrl Pts',(59.9871842641414,-4.03165946910082,5.32469977859742));
#22174=CARTESIAN_POINT('Ctrl Pts',(60.6858451039897,-1.63165946910082,5.83183545124052));
#22175=CARTESIAN_POINT('Ctrl Pts',(60.6858451039897,-4.03165946910082,5.83183545124052));
#22176=CARTESIAN_POINT('Ctrl Pts',(61.3291075829706,-1.63165946910082,6.30568784052758));
#22177=CARTESIAN_POINT('Ctrl Pts',(61.3291075829706,-4.03165946910082,6.30568784052758));
#22178=CARTESIAN_POINT('Ctrl Pts',(61.9129286688635,-1.63165946910082,6.72264590044013));
#22179=CARTESIAN_POINT('Ctrl Pts',(61.9129286688635,-4.03165946910082,6.72264590044013));
#22180=CARTESIAN_POINT('Ctrl Pts',(62.4378966914009,-1.63165946910082,7.06401270956655));
#22181=CARTESIAN_POINT('Ctrl Pts',(62.4378966914009,-4.03165946910082,7.06401270956655));
#22182=CARTESIAN_POINT('Ctrl Pts',(62.9110626727188,-1.63165946910082,7.32028203996567));
#22183=CARTESIAN_POINT('Ctrl Pts',(62.9110626727188,-4.03165946910082,7.32028203996567));
#22184=CARTESIAN_POINT('Ctrl Pts',(63.3480382061253,-1.63165946910082,7.49580221124892));
#22185=CARTESIAN_POINT('Ctrl Pts',(63.3480382061253,-4.03165946910082,7.49580221124892));
#22186=CARTESIAN_POINT('Ctrl Pts',(63.7742575841079,-1.63165946910082,7.61203807956635));
#22187=CARTESIAN_POINT('Ctrl Pts',(63.7742575841079,-4.03165946910082,7.61203807956635));
#22188=CARTESIAN_POINT('Ctrl Pts',(64.2192519841205,-1.63165946910082,7.69914552267219));
#22189=CARTESIAN_POINT('Ctrl Pts',(64.2192519841205,-4.03165946910082,7.69914552267219));
#22190=CARTESIAN_POINT('Ctrl Pts',(64.712086468945,-1.63165946910082,7.78936630198725));
#22191=CARTESIAN_POINT('Ctrl Pts',(64.712086468945,-4.03165946910082,7.78936630198725));
#22192=CARTESIAN_POINT('Ctrl Pts',(65.2754113430736,-1.63165946910082,7.90844857460236));
#22193=CARTESIAN_POINT('Ctrl Pts',(65.2754113430736,-4.03165946910082,7.90844857460236));
#22194=CARTESIAN_POINT('Ctrl Pts',(65.9237039528771,-1.63165946910082,8.07283920347654));
#22195=CARTESIAN_POINT('Ctrl Pts',(65.9237039528771,-4.03165946910082,8.07283920347654));
#22196=CARTESIAN_POINT('Ctrl Pts',(66.6557369297143,-1.63165946910082,8.28958012503506));
#22197=CARTESIAN_POINT('Ctrl Pts',(66.6557369297143,-4.03165946910082,8.28958012503506));
#22198=CARTESIAN_POINT('Ctrl Pts',(67.3150092482541,-1.63165946910082,8.50886642156035));
#22199=CARTESIAN_POINT('Ctrl Pts',(67.3150092482541,-4.03165946910082,8.50886642156035));
#22200=CARTESIAN_POINT('Ctrl Pts',(67.8492602326033,-1.63165946910082,8.69890399191606));
#22201=CARTESIAN_POINT('Ctrl Pts',(67.8492602326033,-4.03165946910082,8.69890399191606));
#22202=CARTESIAN_POINT('Ctrl Pts',(68.2198703338295,-1.63165946910082,8.83566471550562));
#22203=CARTESIAN_POINT('Ctrl Pts',(68.2198703338295,-4.03165946910082,8.83566471550562));
#22204=CARTESIAN_POINT('Ctrl Pts',(68.403087843053,-1.63165946910082,8.90436665637972));
#22205=CARTESIAN_POINT('Ctrl Pts',(68.403087843053,-4.03165946910082,8.90436665637972));
#22206=CARTESIAN_POINT('',(34.5886335096989,-1.63165946910082,1.82713536652871));
#22207=CARTESIAN_POINT('Origin',(32.143405418954,-1.63165946910082,3.2164639050219));
#22208=CARTESIAN_POINT('',(30.067343367632,-1.63165946910082,1.31927109386626));
#22209=CARTESIAN_POINT('Origin',(25.6749565963595,-1.63165946910082,-3.12914171551276));
#22210=CARTESIAN_POINT('',(25.3459666144763,-1.63165946910082,3.11371049024365));
#22211=CARTESIAN_POINT('Origin',(24.7143466872546,-1.63165946910082,5.90470262206354));
#23563=UNCERTAINTY_MEASURE_WITH_UNIT(LENGTH_MEASURE(0.01),#23578,
'DISTANCE_ACCURACY_VALUE',
'Maximum model space distance between geometric entities at asserted c
onnectivities');
#23566=UNCERTAINTY_MEASURE_WITH_UNIT(LENGTH_MEASURE(0.01),#23578,
'DISTANCE_ACCURACY_VALUE',
'Maximum model space distance between geometric entities at asserted c
onnectivities');
#23574=(
GEOMETRIC_REPRESENTATION_CONTEXT(3)
GLOBAL_UNCERTAINTY_ASSIGNED_CONTEXT((#23563))
GLOBAL_UNIT_ASSIGNED_CONTEXT((#23578,#23580,#23581))
REPRESENTATION_CONTEXT('','3D')
);
#23577=(
GEOMETRIC_REPRESENTATION_CONTEXT(3)
GLOBAL_UNCERTAINTY_ASSIGNED_CONTEXT((#23566))
GLOBAL_UNIT_ASSIGNED_CONTEXT((#23578,#23580,#23581))
REPRESENTATION_CONTEXT('','3D')
);
#23578=(
LENGTH_UNIT()
NAMED_UNIT(*)
SI_UNIT(.MILLI.,.METRE.)
);
#23580=(
NAMED_UNIT(*)
PLANE_ANGLE_UNIT()
SI_UNIT($,.RADIAN.)
);
#23581=(
NAMED_UNIT(*)
SI_UNIT($,.STERADIAN.)
SOLID_ANGLE_UNIT()
);
#23589=SHAPE_DEFINITION_REPRESENTATION(#23599,#23618);
#23599=PRODUCT_DEFINITION_SHAPE('',$,#23629);
#23618=SHAPE_REPRESENTATION('',(#4485),#23574);
#23621=PRODUCT_DEFINITION_CONTEXT('part definition',#23653,'design');
#23629=PRODUCT_DEFINITION('Clamp_01','Clamp_01',#23639,#23621);
#23639=PRODUCT_DEFINITION_FORMATION('',$,#23662);
#23653=APPLICATION_CONTEXT(
'Core Data for Automotive Mechanical Design Process');
#23654=PRODUCT_CONTEXT('part definition',#23653,'mechanical');
#23662=PRODUCT('Clamp_01','Clamp_01',$,(#23654));
#23668=PRESENTATION_STYLE_ASSIGNMENT((#23673));
#23673=SURFACE_STYLE_USAGE(.BOTH.,#23678);
#23678=SURFACE_SIDE_STYLE('',(#23683));
#23683=SURFACE_STYLE_FILL_AREA(#23688);
#23688=FILL_AREA_STYLE('Opaque(222,222,222)',(#23693));
#23693=FILL_AREA_STYLE_COLOUR('Opaque(222,222,222)',#23698);
#23698=COLOUR_RGB('Opaque(222,222,222)', 0.09019608, 0.27058824, 0.51372549);
ENDSEC;
END-ISO-10303-21;
